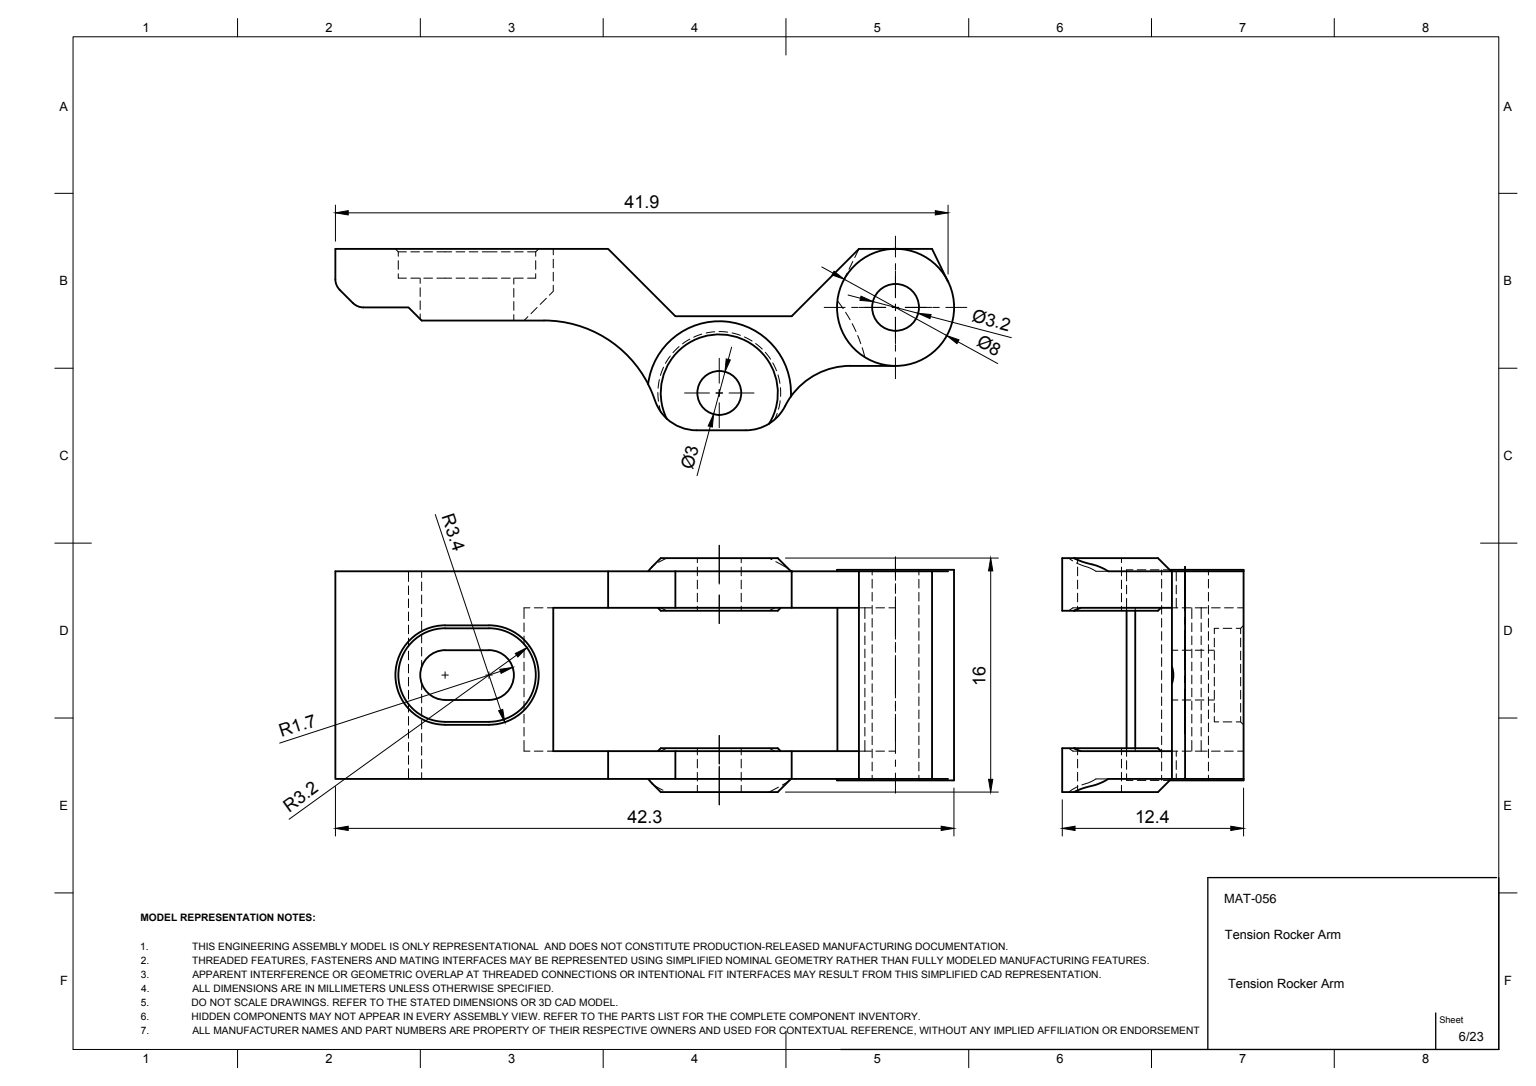
ISO-10303-21;
HEADER;
/* Generated by software containing ST-Developer
 * from STEP Tools, Inc. (www.steptools.com) 
 */

FILE_DESCRIPTION(
/* description */ (''),
/* implementation_level */ '2;1');

FILE_NAME(
/* name */ 'Tension Rocker Arm.step',
/* time_stamp */ '2026-10-28T16:47:13+01:00',
/* author */ (''),
/* organization */ (''),
/* preprocessor_version */ 'ST-DEVELOPER v20.2',
/* originating_system */ 'Autodesk Translation Framework v15.17.0.0',
/* authorisation */ '');

FILE_SCHEMA (('AUTOMOTIVE_DESIGN { 1 0 10303 214 3 1 1 }'));
ENDSEC;

DATA;
#10=MECHANICAL_DESIGN_GEOMETRIC_PRESENTATION_REPRESENTATION('',(#4571),#459242);
#185=ELLIPSE('',#97153,2.40416305603427,1.7);
#4408=SHAPE_REPRESENTATION_RELATIONSHIP('SRR','None',#459333,#4429);
#4429=ADVANCED_BREP_SHAPE_REPRESENTATION('',(#4451),#459222);
#4451=MANIFOLD_SOLID_BREP('Rocker',#94629);
#4571=STYLED_ITEM('',(#459519),#4451);
#4702=CONICAL_SURFACE('',#97156,3.3,0.785398163397448);
#4703=CONICAL_SURFACE('',#97159,3.3,0.785398163397448);
#4704=CONICAL_SURFACE('',#97173,4.45,0.785398163397448);
#4705=CONICAL_SURFACE('',#97175,4.45,0.785398163397449);
#4706=CONICAL_SURFACE('',#97185,4.1,0.785398163397445);
#4707=CONICAL_SURFACE('',#97187,4.1,0.785398163397445);
#5162=FACE_BOUND('',#13230,.T.);
#5163=FACE_BOUND('',#13257,.T.);
#5164=FACE_BOUND('',#13264,.T.);
#5165=FACE_BOUND('',#13266,.T.);
#5166=FACE_BOUND('',#13270,.T.);
#5167=FACE_BOUND('',#13272,.T.);
#5168=FACE_BOUND('',#13278,.T.);
#5169=FACE_BOUND('',#13281,.T.);
#5547=PLANE('',#97094);
#5548=PLANE('',#97095);
#5549=PLANE('',#97096);
#5550=PLANE('',#97103);
#5551=PLANE('',#97112);
#5552=PLANE('',#97113);
#5553=PLANE('',#97122);
#5554=PLANE('',#97123);
#5555=PLANE('',#97127);
#5556=PLANE('',#97130);
#5557=PLANE('',#97131);
#5558=PLANE('',#97134);
#5559=PLANE('',#97136);
#5560=PLANE('',#97137);
#5561=PLANE('',#97138);
#5562=PLANE('',#97139);
#5563=PLANE('',#97143);
#5564=PLANE('',#97144);
#5565=PLANE('',#97151);
#5566=PLANE('',#97152);
#5567=PLANE('',#97158);
#5568=PLANE('',#97161);
#5569=PLANE('',#97162);
#5570=PLANE('',#97165);
#5571=PLANE('',#97168);
#5572=PLANE('',#97170);
#5573=PLANE('',#97171);
#5574=PLANE('',#97177);
#5575=PLANE('',#97181);
#5576=PLANE('',#97189);
#5577=PLANE('',#97193);
#5578=PLANE('',#97199);
#5579=PLANE('',#97201);
#5580=PLANE('',#97204);
#5581=PLANE('',#97206);
#5582=PLANE('',#97209);
#5583=PLANE('',#97211);
#5584=PLANE('',#97212);
#5585=PLANE('',#97218);
#5586=PLANE('',#97219);
#7364=FACE_OUTER_BOUND('',#13221,.T.);
#7365=FACE_OUTER_BOUND('',#13222,.T.);
#7366=FACE_OUTER_BOUND('',#13223,.T.);
#7367=FACE_OUTER_BOUND('',#13224,.T.);
#7368=FACE_OUTER_BOUND('',#13225,.T.);
#7369=FACE_OUTER_BOUND('',#13226,.T.);
#7370=FACE_OUTER_BOUND('',#13227,.T.);
#7371=FACE_OUTER_BOUND('',#13228,.T.);
#7372=FACE_OUTER_BOUND('',#13229,.T.);
#7373=FACE_OUTER_BOUND('',#13231,.T.);
#7374=FACE_OUTER_BOUND('',#13232,.T.);
#7375=FACE_OUTER_BOUND('',#13233,.T.);
#7376=FACE_OUTER_BOUND('',#13234,.T.);
#7377=FACE_OUTER_BOUND('',#13235,.T.);
#7378=FACE_OUTER_BOUND('',#13236,.T.);
#7379=FACE_OUTER_BOUND('',#13237,.T.);
#7380=FACE_OUTER_BOUND('',#13238,.T.);
#7381=FACE_OUTER_BOUND('',#13239,.T.);
#7382=FACE_OUTER_BOUND('',#13240,.T.);
#7383=FACE_OUTER_BOUND('',#13241,.T.);
#7384=FACE_OUTER_BOUND('',#13242,.T.);
#7385=FACE_OUTER_BOUND('',#13243,.T.);
#7386=FACE_OUTER_BOUND('',#13244,.T.);
#7387=FACE_OUTER_BOUND('',#13245,.T.);
#7388=FACE_OUTER_BOUND('',#13246,.T.);
#7389=FACE_OUTER_BOUND('',#13247,.T.);
#7390=FACE_OUTER_BOUND('',#13248,.T.);
#7391=FACE_OUTER_BOUND('',#13249,.T.);
#7392=FACE_OUTER_BOUND('',#13250,.T.);
#7393=FACE_OUTER_BOUND('',#13251,.T.);
#7394=FACE_OUTER_BOUND('',#13252,.T.);
#7395=FACE_OUTER_BOUND('',#13253,.T.);
#7396=FACE_OUTER_BOUND('',#13254,.T.);
#7397=FACE_OUTER_BOUND('',#13255,.T.);
#7398=FACE_OUTER_BOUND('',#13256,.T.);
#7399=FACE_OUTER_BOUND('',#13258,.T.);
#7400=FACE_OUTER_BOUND('',#13259,.T.);
#7401=FACE_OUTER_BOUND('',#13260,.T.);
#7402=FACE_OUTER_BOUND('',#13261,.T.);
#7403=FACE_OUTER_BOUND('',#13262,.T.);
#7404=FACE_OUTER_BOUND('',#13263,.T.);
#7405=FACE_OUTER_BOUND('',#13265,.T.);
#7406=FACE_OUTER_BOUND('',#13267,.T.);
#7407=FACE_OUTER_BOUND('',#13268,.T.);
#7408=FACE_OUTER_BOUND('',#13269,.T.);
#7409=FACE_OUTER_BOUND('',#13271,.T.);
#7410=FACE_OUTER_BOUND('',#13273,.T.);
#7411=FACE_OUTER_BOUND('',#13274,.T.);
#7412=FACE_OUTER_BOUND('',#13275,.T.);
#7413=FACE_OUTER_BOUND('',#13276,.T.);
#7414=FACE_OUTER_BOUND('',#13277,.T.);
#7415=FACE_OUTER_BOUND('',#13279,.T.);
#7416=FACE_OUTER_BOUND('',#13280,.T.);
#7417=FACE_OUTER_BOUND('',#13282,.T.);
#7418=FACE_OUTER_BOUND('',#13283,.T.);
#7419=FACE_OUTER_BOUND('',#13284,.T.);
#7420=FACE_OUTER_BOUND('',#13285,.T.);
#7421=FACE_OUTER_BOUND('',#13286,.T.);
#7422=FACE_OUTER_BOUND('',#13287,.T.);
#7423=FACE_OUTER_BOUND('',#13288,.T.);
#7424=FACE_OUTER_BOUND('',#13289,.T.);
#7425=FACE_OUTER_BOUND('',#13290,.T.);
#7426=FACE_OUTER_BOUND('',#13291,.T.);
#7427=FACE_OUTER_BOUND('',#13292,.T.);
#7428=FACE_OUTER_BOUND('',#13293,.T.);
#7429=FACE_OUTER_BOUND('',#13294,.T.);
#13221=EDGE_LOOP('',(#63426,#63427,#63428,#63429));
#13222=EDGE_LOOP('',(#63430,#63431,#63432,#63433));
#13223=EDGE_LOOP('',(#63434,#63435,#63436,#63437,#63438,#63439,#63440,#63441,
#63442,#63443,#63444,#63445,#63446,#63447,#63448,#63449,#63450));
#13224=EDGE_LOOP('',(#63451,#63452,#63453,#63454,#63455,#63456,#63457,#63458,
#63459,#63460,#63461,#63462,#63463,#63464,#63465,#63466,#63467));
#13225=EDGE_LOOP('',(#63468,#63469,#63470,#63471));
#13226=EDGE_LOOP('',(#63472,#63473,#63474,#63475,#63476,#63477,#63478,#63479,
#63480,#63481,#63482,#63483,#63484,#63485,#63486,#63487,#63488));
#13227=EDGE_LOOP('',(#63489,#63490,#63491,#63492));
#13228=EDGE_LOOP('',(#63493,#63494,#63495,#63496,#63497,#63498,#63499,#63500,
#63501,#63502,#63503,#63504,#63505,#63506));
#13229=EDGE_LOOP('',(#63507,#63508,#63509,#63510,#63511,#63512,#63513,#63514));
#13230=EDGE_LOOP('',(#63515,#63516,#63517,#63518));
#13231=EDGE_LOOP('',(#63519,#63520,#63521,#63522));
#13232=EDGE_LOOP('',(#63523,#63524,#63525,#63526));
#13233=EDGE_LOOP('',(#63527,#63528,#63529,#63530,#63531));
#13234=EDGE_LOOP('',(#63532,#63533,#63534,#63535));
#13235=EDGE_LOOP('',(#63536,#63537,#63538,#63539));
#13236=EDGE_LOOP('',(#63540,#63541,#63542,#63543));
#13237=EDGE_LOOP('',(#63544,#63545,#63546,#63547));
#13238=EDGE_LOOP('',(#63548,#63549,#63550,#63551));
#13239=EDGE_LOOP('',(#63552,#63553,#63554,#63555));
#13240=EDGE_LOOP('',(#63556,#63557,#63558,#63559,#63560,#63561,#63562,#63563,
#63564,#63565));
#13241=EDGE_LOOP('',(#63566,#63567,#63568,#63569));
#13242=EDGE_LOOP('',(#63570,#63571,#63572,#63573));
#13243=EDGE_LOOP('',(#63574,#63575,#63576,#63577,#63578,#63579,#63580,#63581,
#63582,#63583,#63584,#63585,#63586,#63587,#63588,#63589,#63590));
#13244=EDGE_LOOP('',(#63591,#63592,#63593,#63594));
#13245=EDGE_LOOP('',(#63595,#63596,#63597,#63598));
#13246=EDGE_LOOP('',(#63599,#63600,#63601,#63602,#63603,#63604));
#13247=EDGE_LOOP('',(#63605,#63606,#63607,#63608,#63609,#63610));
#13248=EDGE_LOOP('',(#63611,#63612,#63613,#63614));
#13249=EDGE_LOOP('',(#63615,#63616,#63617,#63618));
#13250=EDGE_LOOP('',(#63619,#63620,#63621,#63622));
#13251=EDGE_LOOP('',(#63623,#63624,#63625,#63626));
#13252=EDGE_LOOP('',(#63627,#63628,#63629,#63630));
#13253=EDGE_LOOP('',(#63631,#63632,#63633,#63634));
#13254=EDGE_LOOP('',(#63635,#63636,#63637,#63638));
#13255=EDGE_LOOP('',(#63639,#63640,#63641,#63642));
#13256=EDGE_LOOP('',(#63643,#63644,#63645,#63646));
#13257=EDGE_LOOP('',(#63647,#63648,#63649,#63650));
#13258=EDGE_LOOP('',(#63651,#63652,#63653,#63654));
#13259=EDGE_LOOP('',(#63655,#63656,#63657,#63658));
#13260=EDGE_LOOP('',(#63659,#63660,#63661,#63662));
#13261=EDGE_LOOP('',(#63663,#63664,#63665,#63666,#63667,#63668));
#13262=EDGE_LOOP('',(#63669,#63670,#63671,#63672,#63673,#63674));
#13263=EDGE_LOOP('',(#63675,#63676,#63677,#63678));
#13264=EDGE_LOOP('',(#63679));
#13265=EDGE_LOOP('',(#63680,#63681,#63682,#63683));
#13266=EDGE_LOOP('',(#63684));
#13267=EDGE_LOOP('',(#63685,#63686,#63687,#63688));
#13268=EDGE_LOOP('',(#63689,#63690,#63691,#63692));
#13269=EDGE_LOOP('',(#63693,#63694,#63695,#63696));
#13270=EDGE_LOOP('',(#63697));
#13271=EDGE_LOOP('',(#63698,#63699,#63700,#63701));
#13272=EDGE_LOOP('',(#63702));
#13273=EDGE_LOOP('',(#63703,#63704,#63705,#63706,#63707));
#13274=EDGE_LOOP('',(#63708,#63709,#63710,#63711,#63712,#63713,#63714));
#13275=EDGE_LOOP('',(#63715,#63716,#63717,#63718));
#13276=EDGE_LOOP('',(#63719,#63720,#63721,#63722,#63723,#63724,#63725));
#13277=EDGE_LOOP('',(#63726));
#13278=EDGE_LOOP('',(#63727));
#13279=EDGE_LOOP('',(#63728,#63729,#63730));
#13280=EDGE_LOOP('',(#63731));
#13281=EDGE_LOOP('',(#63732));
#13282=EDGE_LOOP('',(#63733,#63734,#63735));
#13283=EDGE_LOOP('',(#63736,#63737,#63738,#63739));
#13284=EDGE_LOOP('',(#63740,#63741,#63742,#63743));
#13285=EDGE_LOOP('',(#63744,#63745,#63746,#63747,#63748));
#13286=EDGE_LOOP('',(#63749,#63750,#63751,#63752,#63753));
#13287=EDGE_LOOP('',(#63754,#63755,#63756,#63757,#63758,#63759,#63760));
#13288=EDGE_LOOP('',(#63761,#63762,#63763,#63764));
#13289=EDGE_LOOP('',(#63765,#63766,#63767,#63768,#63769,#63770,#63771));
#13290=EDGE_LOOP('',(#63772,#63773,#63774,#63775));
#13291=EDGE_LOOP('',(#63776,#63777,#63778,#63779));
#13292=EDGE_LOOP('',(#63780,#63781,#63782,#63783));
#13293=EDGE_LOOP('',(#63784,#63785,#63786,#63787));
#13294=EDGE_LOOP('',(#63788,#63789,#63790,#63791,#63792,#63793,#63794,#63795,
#63796,#63797,#63798,#63799,#63800,#63801,#63802,#63803,#63804,#63805));
#19394=CIRCLE('',#97097,4.);
#19395=CIRCLE('',#97098,5.);
#19396=CIRCLE('',#97099,4.9);
#19397=CIRCLE('',#97100,8.);
#19398=CIRCLE('',#97101,1.);
#19399=CIRCLE('',#97102,1.);
#19400=CIRCLE('',#97104,4.);
#19401=CIRCLE('',#97105,10.25);
#19402=CIRCLE('',#97106,4.);
#19403=CIRCLE('',#97107,5.);
#19404=CIRCLE('',#97108,3.);
#19405=CIRCLE('',#97109,4.2);
#19406=CIRCLE('',#97110,3.);
#19407=CIRCLE('',#97111,8.);
#19408=CIRCLE('',#97114,8.);
#19409=CIRCLE('',#97115,3.);
#19410=CIRCLE('',#97116,4.2);
#19411=CIRCLE('',#97117,3.);
#19412=CIRCLE('',#97118,5.);
#19413=CIRCLE('',#97119,4.);
#19414=CIRCLE('',#97120,10.25);
#19415=CIRCLE('',#97121,4.);
#19416=CIRCLE('',#97124,1.7);
#19417=CIRCLE('',#97125,1.7);
#19418=CIRCLE('',#97126,1.7);
#19419=CIRCLE('',#97128,3.4);
#19420=CIRCLE('',#97129,3.4);
#19421=CIRCLE('',#97140,4.);
#19422=CIRCLE('',#97142,1.);
#19423=CIRCLE('',#97145,1.);
#19424=CIRCLE('',#97146,8.);
#19425=CIRCLE('',#97147,4.9);
#19426=CIRCLE('',#97148,5.);
#19427=CIRCLE('',#97149,4.);
#19428=CIRCLE('',#97155,1.7);
#19429=CIRCLE('',#97157,3.2);
#19430=CIRCLE('',#97160,3.2);
#19431=CIRCLE('',#97164,3.2);
#19432=CIRCLE('',#97167,3.2);
#19433=CIRCLE('',#97169,1.7);
#19434=CIRCLE('',#97174,4.);
#19435=CIRCLE('',#97176,4.);
#19436=CIRCLE('',#97178,3.);
#19437=CIRCLE('',#97179,2.99999999999999);
#19438=CIRCLE('',#97180,1.5);
#19439=CIRCLE('',#97182,3.);
#19440=CIRCLE('',#97183,2.99999999999999);
#19441=CIRCLE('',#97184,1.5);
#19442=CIRCLE('',#97186,4.);
#19443=CIRCLE('',#97188,4.);
#19444=CIRCLE('',#97190,2.99999999999999);
#19445=CIRCLE('',#97191,3.);
#19446=CIRCLE('',#97192,1.5);
#19447=CIRCLE('',#97194,3.);
#19448=CIRCLE('',#97195,2.99999999999999);
#19449=CIRCLE('',#97196,1.5);
#19450=CIRCLE('',#97202,4.);
#19451=CIRCLE('',#97203,1.6);
#19452=CIRCLE('',#97205,4.);
#19453=CIRCLE('',#97207,4.);
#19454=CIRCLE('',#97208,1.6);
#19455=CIRCLE('',#97210,4.);
#23745=B_SPLINE_CURVE_WITH_KNOTS('',3,(#145559,#145560,#145561,#145562,
#145563,#145564),.UNSPECIFIED.,.F.,.F.,(4,2,4),(1.70223819819958,1.73108544940882,
1.82543924719591),.UNSPECIFIED.);
#23746=B_SPLINE_CURVE_WITH_KNOTS('',3,(#145675,#145676,#145677,#145678,
#145679,#145680),.UNSPECIFIED.,.F.,.F.,(4,2,4),(3.10863777787119,3.15979788758472,
3.18717384259103),.UNSPECIFIED.);
#23747=B_SPLINE_CURVE_WITH_KNOTS('',3,(#145682,#145683,#145684,#145685,
#145686,#145687),.UNSPECIFIED.,.F.,.F.,(4,2,4),(0.820560587522253,0.903541428390679,
0.986302965827679),.UNSPECIFIED.);
#23748=B_SPLINE_CURVE_WITH_KNOTS('',3,(#145690,#145691,#145692,#145693,
#145694,#145695,#145696,#145697),.UNSPECIFIED.,.F.,.F.,(4,2,2,4),(1.04408314569026,
1.07700516790035,1.159852876147,1.19188777117613),.UNSPECIFIED.);
#23749=B_SPLINE_CURVE_WITH_KNOTS('',3,(#145700,#145701,#145702,#145703,
#145704,#145705),.UNSPECIFIED.,.F.,.F.,(4,2,4),(0.461890211108374,0.489266166114685,
0.540426267783997),.UNSPECIFIED.);
#23750=B_SPLINE_CURVE_WITH_KNOTS('',3,(#145707,#145708,#145709,#145710,
#145711,#145712),.UNSPECIFIED.,.F.,.F.,(4,2,4),(1.94461759101078,2.03897139402255,
2.06781864523179),.UNSPECIFIED.);
#23751=B_SPLINE_CURVE_WITH_KNOTS('',3,(#145714,#145715,#145716,#145717,
#145718,#145719,#145720,#145721),.UNSPECIFIED.,.F.,.F.,(4,2,2,4),(0.734169017530397,
0.766203907566677,0.84905161581333,0.881973638023425),.UNSPECIFIED.);
#23752=B_SPLINE_CURVE_WITH_KNOTS('',3,(#145724,#145725,#145726,#145727,
#145728,#145729),.UNSPECIFIED.,.F.,.F.,(4,2,4),(0.991122094940072,1.07388363237707,
1.15686448098652),.UNSPECIFIED.);
#23753=B_SPLINE_CURVE_WITH_KNOTS('',3,(#145748,#145749,#145750,#145751),
 .UNSPECIFIED.,.F.,.F.,(4,4),(0.938179827022778,0.986302965827679),
 .UNSPECIFIED.);
#23754=B_SPLINE_CURVE_WITH_KNOTS('',3,(#145754,#145755,#145756,#145757,
#145758,#145759),.UNSPECIFIED.,.F.,.F.,(4,2,4),(1.04408314569026,1.07700516790035,
1.10576357261676),.UNSPECIFIED.);
#23755=B_SPLINE_CURVE_WITH_KNOTS('',3,(#145762,#145763,#145764,#145765,
#145766,#145767),.UNSPECIFIED.,.F.,.F.,(4,2,4),(0.820293211096921,0.84905161581333,
0.881973638023425),.UNSPECIFIED.);
#23756=B_SPLINE_CURVE_WITH_KNOTS('',3,(#145770,#145771,#145772,#145773),
 .UNSPECIFIED.,.F.,.F.,(4,4),(0.991122094940074,1.03924523374497),
 .UNSPECIFIED.);
#28169=LINE('',#145402,#31971);
#28170=LINE('',#145404,#31972);
#28171=LINE('',#145406,#31973);
#28172=LINE('',#145407,#31974);
#28173=LINE('',#145411,#31975);
#28174=LINE('',#145413,#31976);
#28175=LINE('',#145415,#31977);
#28176=LINE('',#145416,#31978);
#28177=LINE('',#145419,#31979);
#28178=LINE('',#145421,#31980);
#28179=LINE('',#145425,#31981);
#28180=LINE('',#145433,#31982);
#28181=LINE('',#145435,#31983);
#28182=LINE('',#145437,#31984);
#28183=LINE('',#145441,#31985);
#28184=LINE('',#145445,#31986);
#28185=LINE('',#145447,#31987);
#28186=LINE('',#145448,#31988);
#28187=LINE('',#145451,#31989);
#28188=LINE('',#145453,#31990);
#28189=LINE('',#145461,#31991);
#28190=LINE('',#145473,#31992);
#28191=LINE('',#145475,#31993);
#28192=LINE('',#145477,#31994);
#28193=LINE('',#145479,#31995);
#28194=LINE('',#145480,#31996);
#28195=LINE('',#145482,#31997);
#28196=LINE('',#145484,#31998);
#28197=LINE('',#145485,#31999);
#28198=LINE('',#145488,#32000);
#28199=LINE('',#145490,#32001);
#28200=LINE('',#145492,#32002);
#28201=LINE('',#145494,#32003);
#28202=LINE('',#145496,#32004);
#28203=LINE('',#145498,#32005);
#28204=LINE('',#145510,#32006);
#28205=LINE('',#145517,#32007);
#28206=LINE('',#145518,#32008);
#28207=LINE('',#145521,#32009);
#28208=LINE('',#145523,#32010);
#28209=LINE('',#145525,#32011);
#28210=LINE('',#145529,#32012);
#28211=LINE('',#145533,#32013);
#28212=LINE('',#145536,#32014);
#28213=LINE('',#145537,#32015);
#28214=LINE('',#145539,#32016);
#28215=LINE('',#145540,#32017);
#28216=LINE('',#145542,#32018);
#28217=LINE('',#145544,#32019);
#28218=LINE('',#145545,#32020);
#28219=LINE('',#145550,#32021);
#28220=LINE('',#145553,#32022);
#28221=LINE('',#145555,#32023);
#28222=LINE('',#145565,#32024);
#28223=LINE('',#145567,#32025);
#28224=LINE('',#145569,#32026);
#28225=LINE('',#145570,#32027);
#28226=LINE('',#145572,#32028);
#28227=LINE('',#145575,#32029);
#28228=LINE('',#145576,#32030);
#28229=LINE('',#145578,#32031);
#28230=LINE('',#145582,#32032);
#28231=LINE('',#145584,#32033);
#28232=LINE('',#145586,#32034);
#28233=LINE('',#145588,#32035);
#28234=LINE('',#145590,#32036);
#28235=LINE('',#145596,#32037);
#28236=LINE('',#145597,#32038);
#28237=LINE('',#145600,#32039);
#28238=LINE('',#145601,#32040);
#28239=LINE('',#145604,#32041);
#28240=LINE('',#145607,#32042);
#28241=LINE('',#145608,#32043);
#28242=LINE('',#145616,#32044);
#28243=LINE('',#145619,#32045);
#28244=LINE('',#145621,#32046);
#28245=LINE('',#145626,#32047);
#28246=LINE('',#145629,#32048);
#28247=LINE('',#145632,#32049);
#28248=LINE('',#145634,#32050);
#28249=LINE('',#145638,#32051);
#28250=LINE('',#145639,#32052);
#28251=LINE('',#145642,#32053);
#28252=LINE('',#145645,#32054);
#28253=LINE('',#145648,#32055);
#28254=LINE('',#145650,#32056);
#28255=LINE('',#145651,#32057);
#28256=LINE('',#145654,#32058);
#28257=LINE('',#145658,#32059);
#28258=LINE('',#145659,#32060);
#28259=LINE('',#145664,#32061);
#28260=LINE('',#145667,#32062);
#28261=LINE('',#145669,#32063);
#28262=LINE('',#145671,#32064);
#28263=LINE('',#145733,#32065);
#28264=LINE('',#145742,#32066);
#28265=LINE('',#145777,#32067);
#28266=LINE('',#145787,#32068);
#28267=LINE('',#145791,#32069);
#28268=LINE('',#145793,#32070);
#28269=LINE('',#145794,#32071);
#28270=LINE('',#145796,#32072);
#28271=LINE('',#145806,#32073);
#28272=LINE('',#145815,#32074);
#28273=LINE('',#145817,#32075);
#28274=LINE('',#145818,#32076);
#28275=LINE('',#145820,#32077);
#28276=LINE('',#145821,#32078);
#28277=LINE('',#145824,#32079);
#28278=LINE('',#145827,#32080);
#28279=LINE('',#145831,#32081);
#28280=LINE('',#145833,#32082);
#28281=LINE('',#145835,#32083);
#28282=LINE('',#145837,#32084);
#28283=LINE('',#145838,#32085);
#31971=VECTOR('',#111079,10.);
#31972=VECTOR('',#111080,10.);
#31973=VECTOR('',#111081,10.);
#31974=VECTOR('',#111082,10.);
#31975=VECTOR('',#111085,10.);
#31976=VECTOR('',#111086,10.);
#31977=VECTOR('',#111087,10.);
#31978=VECTOR('',#111088,10.);
#31979=VECTOR('',#111091,10.);
#31980=VECTOR('',#111092,10.);
#31981=VECTOR('',#111095,10.);
#31982=VECTOR('',#111102,10.);
#31983=VECTOR('',#111103,10.);
#31984=VECTOR('',#111104,10.);
#31985=VECTOR('',#111107,10.);
#31986=VECTOR('',#111110,10.);
#31987=VECTOR('',#111111,10.);
#31988=VECTOR('',#111112,10.);
#31989=VECTOR('',#111115,10.);
#31990=VECTOR('',#111116,10.);
#31991=VECTOR('',#111123,10.);
#31992=VECTOR('',#111134,10.);
#31993=VECTOR('',#111135,10.);
#31994=VECTOR('',#111136,10.);
#31995=VECTOR('',#111137,10.);
#31996=VECTOR('',#111138,10.);
#31997=VECTOR('',#111141,10.);
#31998=VECTOR('',#111142,10.);
#31999=VECTOR('',#111143,10.);
#32000=VECTOR('',#111146,10.);
#32001=VECTOR('',#111147,10.);
#32002=VECTOR('',#111148,10.);
#32003=VECTOR('',#111149,10.);
#32004=VECTOR('',#111150,10.);
#32005=VECTOR('',#111151,10.);
#32006=VECTOR('',#111162,10.);
#32007=VECTOR('',#111171,10.);
#32008=VECTOR('',#111172,10.);
#32009=VECTOR('',#111175,8.);
#32010=VECTOR('',#111176,10.);
#32011=VECTOR('',#111177,10.);
#32012=VECTOR('',#111180,10.);
#32013=VECTOR('',#111183,10.);
#32014=VECTOR('',#111186,10.);
#32015=VECTOR('',#111187,8.);
#32016=VECTOR('',#111190,10.);
#32017=VECTOR('',#111191,10.);
#32018=VECTOR('',#111192,10.);
#32019=VECTOR('',#111193,10.);
#32020=VECTOR('',#111194,10.);
#32021=VECTOR('',#111197,10.);
#32022=VECTOR('',#111200,10.);
#32023=VECTOR('',#111203,10.);
#32024=VECTOR('',#111208,10.);
#32025=VECTOR('',#111211,10.);
#32026=VECTOR('',#111214,5.);
#32027=VECTOR('',#111215,10.);
#32028=VECTOR('',#111218,10.);
#32029=VECTOR('',#111221,10.);
#32030=VECTOR('',#111222,10.);
#32031=VECTOR('',#111225,10.);
#32032=VECTOR('',#111230,10.);
#32033=VECTOR('',#111231,10.);
#32034=VECTOR('',#111232,10.);
#32035=VECTOR('',#111233,10.);
#32036=VECTOR('',#111234,10.);
#32037=VECTOR('',#111241,10.);
#32038=VECTOR('',#111242,10.);
#32039=VECTOR('',#111245,10.);
#32040=VECTOR('',#111246,10.);
#32041=VECTOR('',#111249,10.);
#32042=VECTOR('',#111252,10.);
#32043=VECTOR('',#111253,10.);
#32044=VECTOR('',#111260,10.);
#32045=VECTOR('',#111265,10.);
#32046=VECTOR('',#111268,10.);
#32047=VECTOR('',#111275,10.);
#32048=VECTOR('',#111278,10.);
#32049=VECTOR('',#111281,10.);
#32050=VECTOR('',#111282,10.);
#32051=VECTOR('',#111287,10.);
#32052=VECTOR('',#111288,10.);
#32053=VECTOR('',#111291,10.);
#32054=VECTOR('',#111296,10.);
#32055=VECTOR('',#111299,10.);
#32056=VECTOR('',#111300,10.);
#32057=VECTOR('',#111301,10.);
#32058=VECTOR('',#111304,10.);
#32059=VECTOR('',#111309,10.);
#32060=VECTOR('',#111310,10.);
#32061=VECTOR('',#111317,10.);
#32062=VECTOR('',#111320,10.);
#32063=VECTOR('',#111323,10.);
#32064=VECTOR('',#111326,10.);
#32065=VECTOR('',#111339,10.);
#32066=VECTOR('',#111350,10.);
#32067=VECTOR('',#111365,10.);
#32068=VECTOR('',#111378,10.);
#32069=VECTOR('',#111383,10.);
#32070=VECTOR('',#111386,10.);
#32071=VECTOR('',#111387,10.);
#32072=VECTOR('',#111390,10.);
#32073=VECTOR('',#111403,10.);
#32074=VECTOR('',#111414,10.);
#32075=VECTOR('',#111417,10.);
#32076=VECTOR('',#111418,5.);
#32077=VECTOR('',#111421,10.);
#32078=VECTOR('',#111422,10.);
#32079=VECTOR('',#111427,10.);
#32080=VECTOR('',#111432,1.5);
#32081=VECTOR('',#111439,10.);
#32082=VECTOR('',#111442,1.6);
#32083=VECTOR('',#111445,1.5);
#32084=VECTOR('',#111448,4.);
#32085=VECTOR('',#111449,4.);
#36364=VERTEX_POINT('',#145400);
#36365=VERTEX_POINT('',#145401);
#36366=VERTEX_POINT('',#145403);
#36367=VERTEX_POINT('',#145405);
#36368=VERTEX_POINT('',#145409);
#36369=VERTEX_POINT('',#145410);
#36370=VERTEX_POINT('',#145412);
#36371=VERTEX_POINT('',#145414);
#36372=VERTEX_POINT('',#145418);
#36373=VERTEX_POINT('',#145420);
#36374=VERTEX_POINT('',#145422);
#36375=VERTEX_POINT('',#145424);
#36376=VERTEX_POINT('',#145426);
#36377=VERTEX_POINT('',#145428);
#36378=VERTEX_POINT('',#145430);
#36379=VERTEX_POINT('',#145432);
#36380=VERTEX_POINT('',#145434);
#36381=VERTEX_POINT('',#145436);
#36382=VERTEX_POINT('',#145438);
#36383=VERTEX_POINT('',#145440);
#36384=VERTEX_POINT('',#145442);
#36385=VERTEX_POINT('',#145444);
#36386=VERTEX_POINT('',#145446);
#36387=VERTEX_POINT('',#145450);
#36388=VERTEX_POINT('',#145452);
#36389=VERTEX_POINT('',#145454);
#36390=VERTEX_POINT('',#145456);
#36391=VERTEX_POINT('',#145458);
#36392=VERTEX_POINT('',#145460);
#36393=VERTEX_POINT('',#145462);
#36394=VERTEX_POINT('',#145464);
#36395=VERTEX_POINT('',#145466);
#36396=VERTEX_POINT('',#145468);
#36397=VERTEX_POINT('',#145470);
#36398=VERTEX_POINT('',#145472);
#36399=VERTEX_POINT('',#145474);
#36400=VERTEX_POINT('',#145476);
#36401=VERTEX_POINT('',#145478);
#36402=VERTEX_POINT('',#145483);
#36403=VERTEX_POINT('',#145487);
#36404=VERTEX_POINT('',#145489);
#36405=VERTEX_POINT('',#145491);
#36406=VERTEX_POINT('',#145493);
#36407=VERTEX_POINT('',#145495);
#36408=VERTEX_POINT('',#145497);
#36409=VERTEX_POINT('',#145499);
#36410=VERTEX_POINT('',#145501);
#36411=VERTEX_POINT('',#145503);
#36412=VERTEX_POINT('',#145505);
#36413=VERTEX_POINT('',#145507);
#36414=VERTEX_POINT('',#145509);
#36415=VERTEX_POINT('',#145511);
#36416=VERTEX_POINT('',#145513);
#36417=VERTEX_POINT('',#145520);
#36418=VERTEX_POINT('',#145522);
#36419=VERTEX_POINT('',#145524);
#36420=VERTEX_POINT('',#145526);
#36421=VERTEX_POINT('',#145528);
#36422=VERTEX_POINT('',#145530);
#36423=VERTEX_POINT('',#145532);
#36424=VERTEX_POINT('',#145534);
#36425=VERTEX_POINT('',#145541);
#36426=VERTEX_POINT('',#145543);
#36427=VERTEX_POINT('',#145546);
#36428=VERTEX_POINT('',#145547);
#36429=VERTEX_POINT('',#145549);
#36430=VERTEX_POINT('',#145551);
#36431=VERTEX_POINT('',#145558);
#36432=VERTEX_POINT('',#145574);
#36433=VERTEX_POINT('',#145581);
#36434=VERTEX_POINT('',#145583);
#36435=VERTEX_POINT('',#145585);
#36436=VERTEX_POINT('',#145587);
#36437=VERTEX_POINT('',#145589);
#36438=VERTEX_POINT('',#145593);
#36439=VERTEX_POINT('',#145594);
#36440=VERTEX_POINT('',#145599);
#36441=VERTEX_POINT('',#145603);
#36442=VERTEX_POINT('',#145606);
#36443=VERTEX_POINT('',#145609);
#36444=VERTEX_POINT('',#145611);
#36445=VERTEX_POINT('',#145613);
#36446=VERTEX_POINT('',#145615);
#36447=VERTEX_POINT('',#145625);
#36448=VERTEX_POINT('',#145627);
#36449=VERTEX_POINT('',#145631);
#36450=VERTEX_POINT('',#145633);
#36451=VERTEX_POINT('',#145637);
#36452=VERTEX_POINT('',#145641);
#36453=VERTEX_POINT('',#145647);
#36454=VERTEX_POINT('',#145649);
#36455=VERTEX_POINT('',#145653);
#36456=VERTEX_POINT('',#145657);
#36457=VERTEX_POINT('',#145663);
#36458=VERTEX_POINT('',#145665);
#36459=VERTEX_POINT('',#145674);
#36460=VERTEX_POINT('',#145681);
#36461=VERTEX_POINT('',#145688);
#36462=VERTEX_POINT('',#145699);
#36463=VERTEX_POINT('',#145706);
#36464=VERTEX_POINT('',#145713);
#36465=VERTEX_POINT('',#145722);
#36466=VERTEX_POINT('',#145731);
#36467=VERTEX_POINT('',#145732);
#36468=VERTEX_POINT('',#145736);
#36469=VERTEX_POINT('',#145739);
#36470=VERTEX_POINT('',#145741);
#36471=VERTEX_POINT('',#145744);
#36472=VERTEX_POINT('',#145747);
#36473=VERTEX_POINT('',#145752);
#36474=VERTEX_POINT('',#145761);
#36475=VERTEX_POINT('',#145768);
#36476=VERTEX_POINT('',#145775);
#36477=VERTEX_POINT('',#145776);
#36478=VERTEX_POINT('',#145780);
#36479=VERTEX_POINT('',#145783);
#36480=VERTEX_POINT('',#145785);
#36481=VERTEX_POINT('',#145788);
#36482=VERTEX_POINT('',#145799);
#36483=VERTEX_POINT('',#145801);
#36484=VERTEX_POINT('',#145804);
#36485=VERTEX_POINT('',#145808);
#36486=VERTEX_POINT('',#145810);
#36487=VERTEX_POINT('',#145813);
#46215=EDGE_CURVE('',#36364,#36365,#28169,.T.);
#46216=EDGE_CURVE('',#36366,#36364,#28170,.T.);
#46217=EDGE_CURVE('',#36367,#36366,#28171,.T.);
#46218=EDGE_CURVE('',#36365,#36367,#28172,.T.);
#46219=EDGE_CURVE('',#36368,#36369,#28173,.T.);
#46220=EDGE_CURVE('',#36370,#36368,#28174,.T.);
#46221=EDGE_CURVE('',#36371,#36370,#28175,.T.);
#46222=EDGE_CURVE('',#36369,#36371,#28176,.T.);
#46223=EDGE_CURVE('',#36372,#36367,#28177,.T.);
#46224=EDGE_CURVE('',#36373,#36366,#28178,.T.);
#46225=EDGE_CURVE('',#36373,#36374,#19394,.T.);
#46226=EDGE_CURVE('',#36374,#36375,#28179,.T.);
#46227=EDGE_CURVE('',#36375,#36376,#19395,.F.);
#46228=EDGE_CURVE('',#36377,#36376,#19396,.T.);
#46229=EDGE_CURVE('',#36377,#36378,#19397,.F.);
#46230=EDGE_CURVE('',#36378,#36379,#28180,.T.);
#46231=EDGE_CURVE('',#36379,#36380,#28181,.T.);
#46232=EDGE_CURVE('',#36380,#36381,#28182,.T.);
#46233=EDGE_CURVE('',#36382,#36381,#19398,.T.);
#46234=EDGE_CURVE('',#36383,#36382,#28183,.T.);
#46235=EDGE_CURVE('',#36384,#36383,#19399,.T.);
#46236=EDGE_CURVE('',#36384,#36385,#28184,.T.);
#46237=EDGE_CURVE('',#36386,#36385,#28185,.T.);
#46238=EDGE_CURVE('',#36386,#36372,#28186,.T.);
#46239=EDGE_CURVE('',#36387,#36368,#28187,.T.);
#46240=EDGE_CURVE('',#36369,#36388,#28188,.T.);
#46241=EDGE_CURVE('',#36389,#36388,#19400,.T.);
#46242=EDGE_CURVE('',#36390,#36389,#19401,.T.);
#46243=EDGE_CURVE('',#36391,#36390,#19402,.T.);
#46244=EDGE_CURVE('',#36392,#36391,#28189,.T.);
#46245=EDGE_CURVE('',#36393,#36392,#19403,.T.);
#46246=EDGE_CURVE('',#36394,#36393,#19404,.T.);
#46247=EDGE_CURVE('',#36395,#36394,#19405,.T.);
#46248=EDGE_CURVE('',#36396,#36395,#19406,.T.);
#46249=EDGE_CURVE('',#36397,#36396,#19407,.T.);
#46250=EDGE_CURVE('',#36397,#36398,#28190,.T.);
#46251=EDGE_CURVE('',#36398,#36399,#28191,.T.);
#46252=EDGE_CURVE('',#36399,#36400,#28192,.T.);
#46253=EDGE_CURVE('',#36401,#36400,#28193,.T.);
#46254=EDGE_CURVE('',#36387,#36401,#28194,.T.);
#46255=EDGE_CURVE('',#36364,#36369,#28195,.T.);
#46256=EDGE_CURVE('',#36364,#36402,#28196,.T.);
#46257=EDGE_CURVE('',#36402,#36388,#28197,.T.);
#46258=EDGE_CURVE('',#36365,#36403,#28198,.T.);
#46259=EDGE_CURVE('',#36404,#36403,#28199,.T.);
#46260=EDGE_CURVE('',#36405,#36404,#28200,.T.);
#46261=EDGE_CURVE('',#36405,#36406,#28201,.T.);
#46262=EDGE_CURVE('',#36407,#36406,#28202,.F.);
#46263=EDGE_CURVE('',#36407,#36408,#28203,.T.);
#46264=EDGE_CURVE('',#36409,#36408,#19408,.T.);
#46265=EDGE_CURVE('',#36410,#36409,#19409,.T.);
#46266=EDGE_CURVE('',#36411,#36410,#19410,.T.);
#46267=EDGE_CURVE('',#36412,#36411,#19411,.T.);
#46268=EDGE_CURVE('',#36413,#36412,#19412,.T.);
#46269=EDGE_CURVE('',#36414,#36413,#28204,.T.);
#46270=EDGE_CURVE('',#36415,#36414,#19413,.T.);
#46271=EDGE_CURVE('',#36416,#36415,#19414,.T.);
#46272=EDGE_CURVE('',#36402,#36416,#19415,.T.);
#46273=EDGE_CURVE('',#36406,#36399,#28205,.T.);
#46274=EDGE_CURVE('',#36398,#36407,#28206,.T.);
#46275=EDGE_CURVE('',#36417,#36397,#28207,.T.);
#46276=EDGE_CURVE('',#36418,#36417,#28208,.F.);
#46277=EDGE_CURVE('',#36418,#36419,#28209,.T.);
#46278=EDGE_CURVE('',#36419,#36420,#19416,.T.);
#46279=EDGE_CURVE('',#36420,#36421,#28210,.T.);
#46280=EDGE_CURVE('',#36421,#36422,#19417,.T.);
#46281=EDGE_CURVE('',#36422,#36423,#28211,.T.);
#46282=EDGE_CURVE('',#36423,#36424,#19418,.T.);
#46283=EDGE_CURVE('',#36424,#36379,#28212,.T.);
#46284=EDGE_CURVE('',#36408,#36378,#28213,.T.);
#46285=EDGE_CURVE('',#36400,#36405,#28214,.T.);
#46286=EDGE_CURVE('',#36404,#36386,#28215,.T.);
#46287=EDGE_CURVE('',#36385,#36425,#28216,.F.);
#46288=EDGE_CURVE('',#36426,#36425,#28217,.F.);
#46289=EDGE_CURVE('',#36426,#36401,#28218,.T.);
#46290=EDGE_CURVE('',#36427,#36428,#19419,.T.);
#46291=EDGE_CURVE('',#36429,#36427,#28219,.T.);
#46292=EDGE_CURVE('',#36430,#36429,#19420,.T.);
#46293=EDGE_CURVE('',#36428,#36430,#28220,.T.);
#46294=EDGE_CURVE('',#36403,#36372,#28221,.T.);
#46295=EDGE_CURVE('',#36377,#36431,#23745,.T.);
#46296=EDGE_CURVE('',#36409,#36431,#28222,.T.);
#46297=EDGE_CURVE('',#36389,#36416,#28223,.T.);
#46298=EDGE_CURVE('',#36375,#36413,#28224,.T.);
#46299=EDGE_CURVE('',#36374,#36414,#28225,.T.);
#46300=EDGE_CURVE('',#36415,#36390,#28226,.T.);
#46301=EDGE_CURVE('',#36432,#36426,#28227,.T.);
#46302=EDGE_CURVE('',#36432,#36387,#28228,.T.);
#46303=EDGE_CURVE('',#36370,#36432,#28229,.T.);
#46304=EDGE_CURVE('',#36433,#36371,#28230,.F.);
#46305=EDGE_CURVE('',#36434,#36433,#28231,.F.);
#46306=EDGE_CURVE('',#36435,#36434,#28232,.F.);
#46307=EDGE_CURVE('',#36436,#36435,#28233,.T.);
#46308=EDGE_CURVE('',#36436,#36437,#28234,.T.);
#46309=EDGE_CURVE('',#36437,#36373,#19421,.T.);
#46310=EDGE_CURVE('',#36438,#36439,#19422,.T.);
#46311=EDGE_CURVE('',#36439,#36382,#28235,.T.);
#46312=EDGE_CURVE('',#36381,#36438,#28236,.T.);
#46313=EDGE_CURVE('',#36439,#36440,#28237,.T.);
#46314=EDGE_CURVE('',#36383,#36440,#28238,.T.);
#46315=EDGE_CURVE('',#36425,#36441,#28239,.T.);
#46316=EDGE_CURVE('',#36440,#36441,#19423,.T.);
#46317=EDGE_CURVE('',#36438,#36442,#28240,.T.);
#46318=EDGE_CURVE('',#36442,#36418,#28241,.T.);
#46319=EDGE_CURVE('',#36443,#36417,#19424,.T.);
#46320=EDGE_CURVE('',#36444,#36443,#19425,.T.);
#46321=EDGE_CURVE('',#36445,#36444,#19426,.T.);
#46322=EDGE_CURVE('',#36445,#36446,#28242,.F.);
#46323=EDGE_CURVE('',#36446,#36433,#19427,.T.);
#46324=EDGE_CURVE('',#36441,#36384,#28243,.T.);
#46325=EDGE_CURVE('',#36442,#36380,#28244,.T.);
#46326=EDGE_CURVE('',#36419,#36424,#185,.T.);
#46327=EDGE_CURVE('',#36447,#36423,#28245,.T.);
#46328=EDGE_CURVE('',#36447,#36448,#19428,.T.);
#46329=EDGE_CURVE('',#36448,#36420,#28246,.T.);
#46330=EDGE_CURVE('',#36449,#36427,#28247,.T.);
#46331=EDGE_CURVE('',#36428,#36450,#28248,.T.);
#46332=EDGE_CURVE('',#36450,#36449,#19429,.T.);
#46333=EDGE_CURVE('',#36451,#36429,#28249,.T.);
#46334=EDGE_CURVE('',#36449,#36451,#28250,.T.);
#46335=EDGE_CURVE('',#36452,#36430,#28251,.T.);
#46336=EDGE_CURVE('',#36451,#36452,#19430,.T.);
#46337=EDGE_CURVE('',#36452,#36450,#28252,.T.);
#46338=EDGE_CURVE('',#36449,#36453,#28253,.T.);
#46339=EDGE_CURVE('',#36453,#36454,#28254,.T.);
#46340=EDGE_CURVE('',#36451,#36454,#28255,.T.);
#46341=EDGE_CURVE('',#36450,#36455,#28256,.T.);
#46342=EDGE_CURVE('',#36455,#36453,#19431,.T.);
#46343=EDGE_CURVE('',#36452,#36456,#28257,.T.);
#46344=EDGE_CURVE('',#36456,#36455,#28258,.T.);
#46345=EDGE_CURVE('',#36454,#36456,#19432,.T.);
#46346=EDGE_CURVE('',#36457,#36447,#28259,.T.);
#46347=EDGE_CURVE('',#36458,#36457,#19433,.T.);
#46348=EDGE_CURVE('',#36448,#36458,#28260,.T.);
#46349=EDGE_CURVE('',#36457,#36422,#28261,.T.);
#46350=EDGE_CURVE('',#36458,#36421,#28262,.T.);
#46351=EDGE_CURVE('',#36376,#36459,#23746,.F.);
#46352=EDGE_CURVE('',#36460,#36459,#23747,.F.);
#46353=EDGE_CURVE('',#36461,#36460,#19434,.T.);
#46354=EDGE_CURVE('',#36431,#36461,#23748,.F.);
#46355=EDGE_CURVE('',#36444,#36462,#23749,.T.);
#46356=EDGE_CURVE('',#36443,#36463,#23750,.F.);
#46357=EDGE_CURVE('',#36464,#36463,#23751,.F.);
#46358=EDGE_CURVE('',#36465,#36464,#19435,.T.);
#46359=EDGE_CURVE('',#36462,#36465,#23752,.F.);
#46360=EDGE_CURVE('',#36466,#36467,#28263,.T.);
#46361=EDGE_CURVE('',#36467,#36461,#19436,.T.);
#46362=EDGE_CURVE('',#36460,#36466,#19437,.T.);
#46363=EDGE_CURVE('',#36468,#36468,#19438,.T.);
#46364=EDGE_CURVE('',#36464,#36469,#19439,.T.);
#46365=EDGE_CURVE('',#36469,#36470,#28264,.T.);
#46366=EDGE_CURVE('',#36470,#36465,#19440,.T.);
#46367=EDGE_CURVE('',#36471,#36471,#19441,.T.);
#46368=EDGE_CURVE('',#36394,#36472,#23753,.T.);
#46369=EDGE_CURVE('',#36473,#36472,#19442,.T.);
#46370=EDGE_CURVE('',#36473,#36395,#23754,.T.);
#46371=EDGE_CURVE('',#36410,#36474,#23755,.T.);
#46372=EDGE_CURVE('',#36475,#36474,#19443,.T.);
#46373=EDGE_CURVE('',#36475,#36411,#23756,.T.);
#46374=EDGE_CURVE('',#36476,#36477,#28265,.T.);
#46375=EDGE_CURVE('',#36477,#36475,#19444,.T.);
#46376=EDGE_CURVE('',#36474,#36476,#19445,.T.);
#46377=EDGE_CURVE('',#36478,#36478,#19446,.T.);
#46378=EDGE_CURVE('',#36479,#36473,#19447,.T.);
#46379=EDGE_CURVE('',#36472,#36480,#19448,.T.);
#46380=EDGE_CURVE('',#36480,#36479,#28266,.T.);
#46381=EDGE_CURVE('',#36481,#36481,#19449,.T.);
#46382=EDGE_CURVE('',#36463,#36396,#28267,.F.);
#46383=EDGE_CURVE('',#36477,#36466,#28268,.T.);
#46384=EDGE_CURVE('',#36459,#36412,#28269,.T.);
#46385=EDGE_CURVE('',#36467,#36476,#28270,.T.);
#46386=EDGE_CURVE('',#36482,#36482,#19450,.T.);
#46387=EDGE_CURVE('',#36483,#36483,#19451,.T.);
#46388=EDGE_CURVE('',#36434,#36484,#19452,.T.);
#46389=EDGE_CURVE('',#36484,#36435,#28271,.F.);
#46390=EDGE_CURVE('',#36485,#36485,#19453,.T.);
#46391=EDGE_CURVE('',#36486,#36486,#19454,.T.);
#46392=EDGE_CURVE('',#36487,#36437,#19455,.T.);
#46393=EDGE_CURVE('',#36436,#36487,#28272,.T.);
#46394=EDGE_CURVE('',#36391,#36446,#28273,.T.);
#46395=EDGE_CURVE('',#36392,#36445,#28274,.T.);
#46396=EDGE_CURVE('',#36470,#36480,#28275,.T.);
#46397=EDGE_CURVE('',#36479,#36469,#28276,.T.);
#46398=EDGE_CURVE('',#36462,#36393,#28277,.F.);
#46399=EDGE_CURVE('',#36478,#36468,#28278,.T.);
#46400=EDGE_CURVE('',#36487,#36484,#28279,.T.);
#46401=EDGE_CURVE('',#36483,#36486,#28280,.T.);
#46402=EDGE_CURVE('',#36471,#36481,#28281,.T.);
#46403=EDGE_CURVE('',#36482,#36434,#28282,.T.);
#46404=EDGE_CURVE('',#36437,#36485,#28283,.T.);
#63426=ORIENTED_EDGE('',*,*,#46215,.F.);
#63427=ORIENTED_EDGE('',*,*,#46216,.F.);
#63428=ORIENTED_EDGE('',*,*,#46217,.F.);
#63429=ORIENTED_EDGE('',*,*,#46218,.F.);
#63430=ORIENTED_EDGE('',*,*,#46219,.F.);
#63431=ORIENTED_EDGE('',*,*,#46220,.F.);
#63432=ORIENTED_EDGE('',*,*,#46221,.F.);
#63433=ORIENTED_EDGE('',*,*,#46222,.F.);
#63434=ORIENTED_EDGE('',*,*,#46223,.T.);
#63435=ORIENTED_EDGE('',*,*,#46217,.T.);
#63436=ORIENTED_EDGE('',*,*,#46224,.F.);
#63437=ORIENTED_EDGE('',*,*,#46225,.T.);
#63438=ORIENTED_EDGE('',*,*,#46226,.T.);
#63439=ORIENTED_EDGE('',*,*,#46227,.T.);
#63440=ORIENTED_EDGE('',*,*,#46228,.F.);
#63441=ORIENTED_EDGE('',*,*,#46229,.T.);
#63442=ORIENTED_EDGE('',*,*,#46230,.T.);
#63443=ORIENTED_EDGE('',*,*,#46231,.T.);
#63444=ORIENTED_EDGE('',*,*,#46232,.T.);
#63445=ORIENTED_EDGE('',*,*,#46233,.F.);
#63446=ORIENTED_EDGE('',*,*,#46234,.F.);
#63447=ORIENTED_EDGE('',*,*,#46235,.F.);
#63448=ORIENTED_EDGE('',*,*,#46236,.T.);
#63449=ORIENTED_EDGE('',*,*,#46237,.F.);
#63450=ORIENTED_EDGE('',*,*,#46238,.T.);
#63451=ORIENTED_EDGE('',*,*,#46239,.T.);
#63452=ORIENTED_EDGE('',*,*,#46219,.T.);
#63453=ORIENTED_EDGE('',*,*,#46240,.T.);
#63454=ORIENTED_EDGE('',*,*,#46241,.F.);
#63455=ORIENTED_EDGE('',*,*,#46242,.F.);
#63456=ORIENTED_EDGE('',*,*,#46243,.F.);
#63457=ORIENTED_EDGE('',*,*,#46244,.F.);
#63458=ORIENTED_EDGE('',*,*,#46245,.F.);
#63459=ORIENTED_EDGE('',*,*,#46246,.F.);
#63460=ORIENTED_EDGE('',*,*,#46247,.F.);
#63461=ORIENTED_EDGE('',*,*,#46248,.F.);
#63462=ORIENTED_EDGE('',*,*,#46249,.F.);
#63463=ORIENTED_EDGE('',*,*,#46250,.T.);
#63464=ORIENTED_EDGE('',*,*,#46251,.T.);
#63465=ORIENTED_EDGE('',*,*,#46252,.T.);
#63466=ORIENTED_EDGE('',*,*,#46253,.F.);
#63467=ORIENTED_EDGE('',*,*,#46254,.F.);
#63468=ORIENTED_EDGE('',*,*,#46240,.F.);
#63469=ORIENTED_EDGE('',*,*,#46255,.F.);
#63470=ORIENTED_EDGE('',*,*,#46256,.T.);
#63471=ORIENTED_EDGE('',*,*,#46257,.T.);
#63472=ORIENTED_EDGE('',*,*,#46258,.T.);
#63473=ORIENTED_EDGE('',*,*,#46259,.F.);
#63474=ORIENTED_EDGE('',*,*,#46260,.F.);
#63475=ORIENTED_EDGE('',*,*,#46261,.T.);
#63476=ORIENTED_EDGE('',*,*,#46262,.F.);
#63477=ORIENTED_EDGE('',*,*,#46263,.T.);
#63478=ORIENTED_EDGE('',*,*,#46264,.F.);
#63479=ORIENTED_EDGE('',*,*,#46265,.F.);
#63480=ORIENTED_EDGE('',*,*,#46266,.F.);
#63481=ORIENTED_EDGE('',*,*,#46267,.F.);
#63482=ORIENTED_EDGE('',*,*,#46268,.F.);
#63483=ORIENTED_EDGE('',*,*,#46269,.F.);
#63484=ORIENTED_EDGE('',*,*,#46270,.F.);
#63485=ORIENTED_EDGE('',*,*,#46271,.F.);
#63486=ORIENTED_EDGE('',*,*,#46272,.F.);
#63487=ORIENTED_EDGE('',*,*,#46256,.F.);
#63488=ORIENTED_EDGE('',*,*,#46215,.T.);
#63489=ORIENTED_EDGE('',*,*,#46262,.T.);
#63490=ORIENTED_EDGE('',*,*,#46273,.T.);
#63491=ORIENTED_EDGE('',*,*,#46251,.F.);
#63492=ORIENTED_EDGE('',*,*,#46274,.T.);
#63493=ORIENTED_EDGE('',*,*,#46263,.F.);
#63494=ORIENTED_EDGE('',*,*,#46274,.F.);
#63495=ORIENTED_EDGE('',*,*,#46250,.F.);
#63496=ORIENTED_EDGE('',*,*,#46275,.F.);
#63497=ORIENTED_EDGE('',*,*,#46276,.F.);
#63498=ORIENTED_EDGE('',*,*,#46277,.T.);
#63499=ORIENTED_EDGE('',*,*,#46278,.T.);
#63500=ORIENTED_EDGE('',*,*,#46279,.T.);
#63501=ORIENTED_EDGE('',*,*,#46280,.T.);
#63502=ORIENTED_EDGE('',*,*,#46281,.T.);
#63503=ORIENTED_EDGE('',*,*,#46282,.T.);
#63504=ORIENTED_EDGE('',*,*,#46283,.T.);
#63505=ORIENTED_EDGE('',*,*,#46230,.F.);
#63506=ORIENTED_EDGE('',*,*,#46284,.F.);
#63507=ORIENTED_EDGE('',*,*,#46253,.T.);
#63508=ORIENTED_EDGE('',*,*,#46285,.T.);
#63509=ORIENTED_EDGE('',*,*,#46260,.T.);
#63510=ORIENTED_EDGE('',*,*,#46286,.T.);
#63511=ORIENTED_EDGE('',*,*,#46237,.T.);
#63512=ORIENTED_EDGE('',*,*,#46287,.T.);
#63513=ORIENTED_EDGE('',*,*,#46288,.F.);
#63514=ORIENTED_EDGE('',*,*,#46289,.T.);
#63515=ORIENTED_EDGE('',*,*,#46290,.F.);
#63516=ORIENTED_EDGE('',*,*,#46291,.F.);
#63517=ORIENTED_EDGE('',*,*,#46292,.F.);
#63518=ORIENTED_EDGE('',*,*,#46293,.F.);
#63519=ORIENTED_EDGE('',*,*,#46259,.T.);
#63520=ORIENTED_EDGE('',*,*,#46294,.T.);
#63521=ORIENTED_EDGE('',*,*,#46238,.F.);
#63522=ORIENTED_EDGE('',*,*,#46286,.F.);
#63523=ORIENTED_EDGE('',*,*,#46273,.F.);
#63524=ORIENTED_EDGE('',*,*,#46261,.F.);
#63525=ORIENTED_EDGE('',*,*,#46285,.F.);
#63526=ORIENTED_EDGE('',*,*,#46252,.F.);
#63527=ORIENTED_EDGE('',*,*,#46264,.T.);
#63528=ORIENTED_EDGE('',*,*,#46284,.T.);
#63529=ORIENTED_EDGE('',*,*,#46229,.F.);
#63530=ORIENTED_EDGE('',*,*,#46295,.T.);
#63531=ORIENTED_EDGE('',*,*,#46296,.F.);
#63532=ORIENTED_EDGE('',*,*,#46257,.F.);
#63533=ORIENTED_EDGE('',*,*,#46272,.T.);
#63534=ORIENTED_EDGE('',*,*,#46297,.F.);
#63535=ORIENTED_EDGE('',*,*,#46241,.T.);
#63536=ORIENTED_EDGE('',*,*,#46269,.T.);
#63537=ORIENTED_EDGE('',*,*,#46298,.F.);
#63538=ORIENTED_EDGE('',*,*,#46226,.F.);
#63539=ORIENTED_EDGE('',*,*,#46299,.T.);
#63540=ORIENTED_EDGE('',*,*,#46297,.T.);
#63541=ORIENTED_EDGE('',*,*,#46271,.T.);
#63542=ORIENTED_EDGE('',*,*,#46300,.T.);
#63543=ORIENTED_EDGE('',*,*,#46242,.T.);
#63544=ORIENTED_EDGE('',*,*,#46254,.T.);
#63545=ORIENTED_EDGE('',*,*,#46289,.F.);
#63546=ORIENTED_EDGE('',*,*,#46301,.F.);
#63547=ORIENTED_EDGE('',*,*,#46302,.T.);
#63548=ORIENTED_EDGE('',*,*,#46303,.F.);
#63549=ORIENTED_EDGE('',*,*,#46220,.T.);
#63550=ORIENTED_EDGE('',*,*,#46239,.F.);
#63551=ORIENTED_EDGE('',*,*,#46302,.F.);
#63552=ORIENTED_EDGE('',*,*,#46223,.F.);
#63553=ORIENTED_EDGE('',*,*,#46294,.F.);
#63554=ORIENTED_EDGE('',*,*,#46258,.F.);
#63555=ORIENTED_EDGE('',*,*,#46218,.T.);
#63556=ORIENTED_EDGE('',*,*,#46222,.T.);
#63557=ORIENTED_EDGE('',*,*,#46304,.F.);
#63558=ORIENTED_EDGE('',*,*,#46305,.F.);
#63559=ORIENTED_EDGE('',*,*,#46306,.F.);
#63560=ORIENTED_EDGE('',*,*,#46307,.F.);
#63561=ORIENTED_EDGE('',*,*,#46308,.T.);
#63562=ORIENTED_EDGE('',*,*,#46309,.T.);
#63563=ORIENTED_EDGE('',*,*,#46224,.T.);
#63564=ORIENTED_EDGE('',*,*,#46216,.T.);
#63565=ORIENTED_EDGE('',*,*,#46255,.T.);
#63566=ORIENTED_EDGE('',*,*,#46310,.T.);
#63567=ORIENTED_EDGE('',*,*,#46311,.T.);
#63568=ORIENTED_EDGE('',*,*,#46233,.T.);
#63569=ORIENTED_EDGE('',*,*,#46312,.T.);
#63570=ORIENTED_EDGE('',*,*,#46311,.F.);
#63571=ORIENTED_EDGE('',*,*,#46313,.T.);
#63572=ORIENTED_EDGE('',*,*,#46314,.F.);
#63573=ORIENTED_EDGE('',*,*,#46234,.T.);
#63574=ORIENTED_EDGE('',*,*,#46303,.T.);
#63575=ORIENTED_EDGE('',*,*,#46301,.T.);
#63576=ORIENTED_EDGE('',*,*,#46288,.T.);
#63577=ORIENTED_EDGE('',*,*,#46315,.T.);
#63578=ORIENTED_EDGE('',*,*,#46316,.F.);
#63579=ORIENTED_EDGE('',*,*,#46313,.F.);
#63580=ORIENTED_EDGE('',*,*,#46310,.F.);
#63581=ORIENTED_EDGE('',*,*,#46317,.T.);
#63582=ORIENTED_EDGE('',*,*,#46318,.T.);
#63583=ORIENTED_EDGE('',*,*,#46276,.T.);
#63584=ORIENTED_EDGE('',*,*,#46319,.F.);
#63585=ORIENTED_EDGE('',*,*,#46320,.F.);
#63586=ORIENTED_EDGE('',*,*,#46321,.F.);
#63587=ORIENTED_EDGE('',*,*,#46322,.T.);
#63588=ORIENTED_EDGE('',*,*,#46323,.T.);
#63589=ORIENTED_EDGE('',*,*,#46304,.T.);
#63590=ORIENTED_EDGE('',*,*,#46221,.T.);
#63591=ORIENTED_EDGE('',*,*,#46235,.T.);
#63592=ORIENTED_EDGE('',*,*,#46314,.T.);
#63593=ORIENTED_EDGE('',*,*,#46316,.T.);
#63594=ORIENTED_EDGE('',*,*,#46324,.T.);
#63595=ORIENTED_EDGE('',*,*,#46312,.F.);
#63596=ORIENTED_EDGE('',*,*,#46232,.F.);
#63597=ORIENTED_EDGE('',*,*,#46325,.F.);
#63598=ORIENTED_EDGE('',*,*,#46317,.F.);
#63599=ORIENTED_EDGE('',*,*,#46326,.F.);
#63600=ORIENTED_EDGE('',*,*,#46277,.F.);
#63601=ORIENTED_EDGE('',*,*,#46318,.F.);
#63602=ORIENTED_EDGE('',*,*,#46325,.T.);
#63603=ORIENTED_EDGE('',*,*,#46231,.F.);
#63604=ORIENTED_EDGE('',*,*,#46283,.F.);
#63605=ORIENTED_EDGE('',*,*,#46326,.T.);
#63606=ORIENTED_EDGE('',*,*,#46282,.F.);
#63607=ORIENTED_EDGE('',*,*,#46327,.F.);
#63608=ORIENTED_EDGE('',*,*,#46328,.T.);
#63609=ORIENTED_EDGE('',*,*,#46329,.T.);
#63610=ORIENTED_EDGE('',*,*,#46278,.F.);
#63611=ORIENTED_EDGE('',*,*,#46330,.T.);
#63612=ORIENTED_EDGE('',*,*,#46290,.T.);
#63613=ORIENTED_EDGE('',*,*,#46331,.T.);
#63614=ORIENTED_EDGE('',*,*,#46332,.T.);
#63615=ORIENTED_EDGE('',*,*,#46333,.T.);
#63616=ORIENTED_EDGE('',*,*,#46291,.T.);
#63617=ORIENTED_EDGE('',*,*,#46330,.F.);
#63618=ORIENTED_EDGE('',*,*,#46334,.T.);
#63619=ORIENTED_EDGE('',*,*,#46335,.T.);
#63620=ORIENTED_EDGE('',*,*,#46292,.T.);
#63621=ORIENTED_EDGE('',*,*,#46333,.F.);
#63622=ORIENTED_EDGE('',*,*,#46336,.T.);
#63623=ORIENTED_EDGE('',*,*,#46331,.F.);
#63624=ORIENTED_EDGE('',*,*,#46293,.T.);
#63625=ORIENTED_EDGE('',*,*,#46335,.F.);
#63626=ORIENTED_EDGE('',*,*,#46337,.T.);
#63627=ORIENTED_EDGE('',*,*,#46334,.F.);
#63628=ORIENTED_EDGE('',*,*,#46338,.T.);
#63629=ORIENTED_EDGE('',*,*,#46339,.T.);
#63630=ORIENTED_EDGE('',*,*,#46340,.F.);
#63631=ORIENTED_EDGE('',*,*,#46332,.F.);
#63632=ORIENTED_EDGE('',*,*,#46341,.T.);
#63633=ORIENTED_EDGE('',*,*,#46342,.T.);
#63634=ORIENTED_EDGE('',*,*,#46338,.F.);
#63635=ORIENTED_EDGE('',*,*,#46337,.F.);
#63636=ORIENTED_EDGE('',*,*,#46343,.T.);
#63637=ORIENTED_EDGE('',*,*,#46344,.T.);
#63638=ORIENTED_EDGE('',*,*,#46341,.F.);
#63639=ORIENTED_EDGE('',*,*,#46336,.F.);
#63640=ORIENTED_EDGE('',*,*,#46340,.T.);
#63641=ORIENTED_EDGE('',*,*,#46345,.T.);
#63642=ORIENTED_EDGE('',*,*,#46343,.F.);
#63643=ORIENTED_EDGE('',*,*,#46342,.F.);
#63644=ORIENTED_EDGE('',*,*,#46344,.F.);
#63645=ORIENTED_EDGE('',*,*,#46345,.F.);
#63646=ORIENTED_EDGE('',*,*,#46339,.F.);
#63647=ORIENTED_EDGE('',*,*,#46328,.F.);
#63648=ORIENTED_EDGE('',*,*,#46346,.F.);
#63649=ORIENTED_EDGE('',*,*,#46347,.F.);
#63650=ORIENTED_EDGE('',*,*,#46348,.F.);
#63651=ORIENTED_EDGE('',*,*,#46346,.T.);
#63652=ORIENTED_EDGE('',*,*,#46327,.T.);
#63653=ORIENTED_EDGE('',*,*,#46281,.F.);
#63654=ORIENTED_EDGE('',*,*,#46349,.F.);
#63655=ORIENTED_EDGE('',*,*,#46348,.T.);
#63656=ORIENTED_EDGE('',*,*,#46350,.T.);
#63657=ORIENTED_EDGE('',*,*,#46279,.F.);
#63658=ORIENTED_EDGE('',*,*,#46329,.F.);
#63659=ORIENTED_EDGE('',*,*,#46347,.T.);
#63660=ORIENTED_EDGE('',*,*,#46349,.T.);
#63661=ORIENTED_EDGE('',*,*,#46280,.F.);
#63662=ORIENTED_EDGE('',*,*,#46350,.F.);
#63663=ORIENTED_EDGE('',*,*,#46295,.F.);
#63664=ORIENTED_EDGE('',*,*,#46228,.T.);
#63665=ORIENTED_EDGE('',*,*,#46351,.T.);
#63666=ORIENTED_EDGE('',*,*,#46352,.F.);
#63667=ORIENTED_EDGE('',*,*,#46353,.F.);
#63668=ORIENTED_EDGE('',*,*,#46354,.F.);
#63669=ORIENTED_EDGE('',*,*,#46355,.F.);
#63670=ORIENTED_EDGE('',*,*,#46320,.T.);
#63671=ORIENTED_EDGE('',*,*,#46356,.T.);
#63672=ORIENTED_EDGE('',*,*,#46357,.F.);
#63673=ORIENTED_EDGE('',*,*,#46358,.F.);
#63674=ORIENTED_EDGE('',*,*,#46359,.F.);
#63675=ORIENTED_EDGE('',*,*,#46360,.T.);
#63676=ORIENTED_EDGE('',*,*,#46361,.T.);
#63677=ORIENTED_EDGE('',*,*,#46353,.T.);
#63678=ORIENTED_EDGE('',*,*,#46362,.T.);
#63679=ORIENTED_EDGE('',*,*,#46363,.T.);
#63680=ORIENTED_EDGE('',*,*,#46358,.T.);
#63681=ORIENTED_EDGE('',*,*,#46364,.T.);
#63682=ORIENTED_EDGE('',*,*,#46365,.T.);
#63683=ORIENTED_EDGE('',*,*,#46366,.T.);
#63684=ORIENTED_EDGE('',*,*,#46367,.T.);
#63685=ORIENTED_EDGE('',*,*,#46368,.T.);
#63686=ORIENTED_EDGE('',*,*,#46369,.F.);
#63687=ORIENTED_EDGE('',*,*,#46370,.T.);
#63688=ORIENTED_EDGE('',*,*,#46247,.T.);
#63689=ORIENTED_EDGE('',*,*,#46371,.T.);
#63690=ORIENTED_EDGE('',*,*,#46372,.F.);
#63691=ORIENTED_EDGE('',*,*,#46373,.T.);
#63692=ORIENTED_EDGE('',*,*,#46266,.T.);
#63693=ORIENTED_EDGE('',*,*,#46374,.T.);
#63694=ORIENTED_EDGE('',*,*,#46375,.T.);
#63695=ORIENTED_EDGE('',*,*,#46372,.T.);
#63696=ORIENTED_EDGE('',*,*,#46376,.T.);
#63697=ORIENTED_EDGE('',*,*,#46377,.T.);
#63698=ORIENTED_EDGE('',*,*,#46378,.T.);
#63699=ORIENTED_EDGE('',*,*,#46369,.T.);
#63700=ORIENTED_EDGE('',*,*,#46379,.T.);
#63701=ORIENTED_EDGE('',*,*,#46380,.T.);
#63702=ORIENTED_EDGE('',*,*,#46381,.T.);
#63703=ORIENTED_EDGE('',*,*,#46249,.T.);
#63704=ORIENTED_EDGE('',*,*,#46382,.F.);
#63705=ORIENTED_EDGE('',*,*,#46356,.F.);
#63706=ORIENTED_EDGE('',*,*,#46319,.T.);
#63707=ORIENTED_EDGE('',*,*,#46275,.T.);
#63708=ORIENTED_EDGE('',*,*,#46267,.T.);
#63709=ORIENTED_EDGE('',*,*,#46373,.F.);
#63710=ORIENTED_EDGE('',*,*,#46375,.F.);
#63711=ORIENTED_EDGE('',*,*,#46383,.T.);
#63712=ORIENTED_EDGE('',*,*,#46362,.F.);
#63713=ORIENTED_EDGE('',*,*,#46352,.T.);
#63714=ORIENTED_EDGE('',*,*,#46384,.T.);
#63715=ORIENTED_EDGE('',*,*,#46385,.F.);
#63716=ORIENTED_EDGE('',*,*,#46360,.F.);
#63717=ORIENTED_EDGE('',*,*,#46383,.F.);
#63718=ORIENTED_EDGE('',*,*,#46374,.F.);
#63719=ORIENTED_EDGE('',*,*,#46265,.T.);
#63720=ORIENTED_EDGE('',*,*,#46296,.T.);
#63721=ORIENTED_EDGE('',*,*,#46354,.T.);
#63722=ORIENTED_EDGE('',*,*,#46361,.F.);
#63723=ORIENTED_EDGE('',*,*,#46385,.T.);
#63724=ORIENTED_EDGE('',*,*,#46376,.F.);
#63725=ORIENTED_EDGE('',*,*,#46371,.F.);
#63726=ORIENTED_EDGE('',*,*,#46386,.T.);
#63727=ORIENTED_EDGE('',*,*,#46387,.T.);
#63728=ORIENTED_EDGE('',*,*,#46388,.T.);
#63729=ORIENTED_EDGE('',*,*,#46389,.T.);
#63730=ORIENTED_EDGE('',*,*,#46306,.T.);
#63731=ORIENTED_EDGE('',*,*,#46390,.T.);
#63732=ORIENTED_EDGE('',*,*,#46391,.T.);
#63733=ORIENTED_EDGE('',*,*,#46392,.T.);
#63734=ORIENTED_EDGE('',*,*,#46308,.F.);
#63735=ORIENTED_EDGE('',*,*,#46393,.T.);
#63736=ORIENTED_EDGE('',*,*,#46244,.T.);
#63737=ORIENTED_EDGE('',*,*,#46394,.T.);
#63738=ORIENTED_EDGE('',*,*,#46322,.F.);
#63739=ORIENTED_EDGE('',*,*,#46395,.F.);
#63740=ORIENTED_EDGE('',*,*,#46396,.F.);
#63741=ORIENTED_EDGE('',*,*,#46365,.F.);
#63742=ORIENTED_EDGE('',*,*,#46397,.F.);
#63743=ORIENTED_EDGE('',*,*,#46380,.F.);
#63744=ORIENTED_EDGE('',*,*,#46268,.T.);
#63745=ORIENTED_EDGE('',*,*,#46384,.F.);
#63746=ORIENTED_EDGE('',*,*,#46351,.F.);
#63747=ORIENTED_EDGE('',*,*,#46227,.F.);
#63748=ORIENTED_EDGE('',*,*,#46298,.T.);
#63749=ORIENTED_EDGE('',*,*,#46245,.T.);
#63750=ORIENTED_EDGE('',*,*,#46395,.T.);
#63751=ORIENTED_EDGE('',*,*,#46321,.T.);
#63752=ORIENTED_EDGE('',*,*,#46355,.T.);
#63753=ORIENTED_EDGE('',*,*,#46398,.T.);
#63754=ORIENTED_EDGE('',*,*,#46246,.T.);
#63755=ORIENTED_EDGE('',*,*,#46398,.F.);
#63756=ORIENTED_EDGE('',*,*,#46359,.T.);
#63757=ORIENTED_EDGE('',*,*,#46366,.F.);
#63758=ORIENTED_EDGE('',*,*,#46396,.T.);
#63759=ORIENTED_EDGE('',*,*,#46379,.F.);
#63760=ORIENTED_EDGE('',*,*,#46368,.F.);
#63761=ORIENTED_EDGE('',*,*,#46377,.F.);
#63762=ORIENTED_EDGE('',*,*,#46399,.T.);
#63763=ORIENTED_EDGE('',*,*,#46363,.F.);
#63764=ORIENTED_EDGE('',*,*,#46399,.F.);
#63765=ORIENTED_EDGE('',*,*,#46248,.T.);
#63766=ORIENTED_EDGE('',*,*,#46370,.F.);
#63767=ORIENTED_EDGE('',*,*,#46378,.F.);
#63768=ORIENTED_EDGE('',*,*,#46397,.T.);
#63769=ORIENTED_EDGE('',*,*,#46364,.F.);
#63770=ORIENTED_EDGE('',*,*,#46357,.T.);
#63771=ORIENTED_EDGE('',*,*,#46382,.T.);
#63772=ORIENTED_EDGE('',*,*,#46324,.F.);
#63773=ORIENTED_EDGE('',*,*,#46315,.F.);
#63774=ORIENTED_EDGE('',*,*,#46287,.F.);
#63775=ORIENTED_EDGE('',*,*,#46236,.F.);
#63776=ORIENTED_EDGE('',*,*,#46389,.F.);
#63777=ORIENTED_EDGE('',*,*,#46400,.F.);
#63778=ORIENTED_EDGE('',*,*,#46393,.F.);
#63779=ORIENTED_EDGE('',*,*,#46307,.T.);
#63780=ORIENTED_EDGE('',*,*,#46387,.F.);
#63781=ORIENTED_EDGE('',*,*,#46401,.T.);
#63782=ORIENTED_EDGE('',*,*,#46391,.F.);
#63783=ORIENTED_EDGE('',*,*,#46401,.F.);
#63784=ORIENTED_EDGE('',*,*,#46367,.F.);
#63785=ORIENTED_EDGE('',*,*,#46402,.T.);
#63786=ORIENTED_EDGE('',*,*,#46381,.F.);
#63787=ORIENTED_EDGE('',*,*,#46402,.F.);
#63788=ORIENTED_EDGE('',*,*,#46386,.F.);
#63789=ORIENTED_EDGE('',*,*,#46403,.T.);
#63790=ORIENTED_EDGE('',*,*,#46305,.T.);
#63791=ORIENTED_EDGE('',*,*,#46323,.F.);
#63792=ORIENTED_EDGE('',*,*,#46394,.F.);
#63793=ORIENTED_EDGE('',*,*,#46243,.T.);
#63794=ORIENTED_EDGE('',*,*,#46300,.F.);
#63795=ORIENTED_EDGE('',*,*,#46270,.T.);
#63796=ORIENTED_EDGE('',*,*,#46299,.F.);
#63797=ORIENTED_EDGE('',*,*,#46225,.F.);
#63798=ORIENTED_EDGE('',*,*,#46309,.F.);
#63799=ORIENTED_EDGE('',*,*,#46404,.T.);
#63800=ORIENTED_EDGE('',*,*,#46390,.F.);
#63801=ORIENTED_EDGE('',*,*,#46404,.F.);
#63802=ORIENTED_EDGE('',*,*,#46392,.F.);
#63803=ORIENTED_EDGE('',*,*,#46400,.T.);
#63804=ORIENTED_EDGE('',*,*,#46388,.F.);
#63805=ORIENTED_EDGE('',*,*,#46403,.F.);
#87504=CYLINDRICAL_SURFACE('',#97132,8.);
#87505=CYLINDRICAL_SURFACE('',#97133,4.);
#87506=CYLINDRICAL_SURFACE('',#97135,10.25);
#87507=CYLINDRICAL_SURFACE('',#97141,1.);
#87508=CYLINDRICAL_SURFACE('',#97150,1.);
#87509=CYLINDRICAL_SURFACE('',#97154,1.7);
#87510=CYLINDRICAL_SURFACE('',#97163,3.2);
#87511=CYLINDRICAL_SURFACE('',#97166,3.2);
#87512=CYLINDRICAL_SURFACE('',#97172,1.7);
#87513=CYLINDRICAL_SURFACE('',#97197,8.);
#87514=CYLINDRICAL_SURFACE('',#97198,3.);
#87515=CYLINDRICAL_SURFACE('',#97200,3.);
#87516=CYLINDRICAL_SURFACE('',#97213,5.);
#87517=CYLINDRICAL_SURFACE('',#97214,5.);
#87518=CYLINDRICAL_SURFACE('',#97215,3.);
#87519=CYLINDRICAL_SURFACE('',#97216,1.5);
#87520=CYLINDRICAL_SURFACE('',#97217,3.);
#87521=CYLINDRICAL_SURFACE('',#97220,1.6);
#87522=CYLINDRICAL_SURFACE('',#97221,1.5);
#87523=CYLINDRICAL_SURFACE('',#97222,4.);
#89828=ADVANCED_FACE('',(#7364),#5547,.F.);
#89829=ADVANCED_FACE('',(#7365),#5548,.F.);
#89830=ADVANCED_FACE('',(#7366),#5549,.F.);
#89831=ADVANCED_FACE('',(#7367),#5550,.F.);
#89832=ADVANCED_FACE('',(#7368),#5551,.T.);
#89833=ADVANCED_FACE('',(#7369),#5552,.T.);
#89834=ADVANCED_FACE('',(#7370),#5553,.T.);
#89835=ADVANCED_FACE('',(#7371),#5554,.T.);
#89836=ADVANCED_FACE('',(#7372,#5162),#5555,.T.);
#89837=ADVANCED_FACE('',(#7373),#5556,.F.);
#89838=ADVANCED_FACE('',(#7374),#5557,.F.);
#89839=ADVANCED_FACE('',(#7375),#87504,.F.);
#89840=ADVANCED_FACE('',(#7376),#87505,.T.);
#89841=ADVANCED_FACE('',(#7377),#5558,.T.);
#89842=ADVANCED_FACE('',(#7378),#87506,.F.);
#89843=ADVANCED_FACE('',(#7379),#5559,.F.);
#89844=ADVANCED_FACE('',(#7380),#5560,.F.);
#89845=ADVANCED_FACE('',(#7381),#5561,.F.);
#89846=ADVANCED_FACE('',(#7382),#5562,.T.);
#89847=ADVANCED_FACE('',(#7383),#87507,.T.);
#89848=ADVANCED_FACE('',(#7384),#5563,.T.);
#89849=ADVANCED_FACE('',(#7385),#5564,.F.);
#89850=ADVANCED_FACE('',(#7386),#87508,.T.);
#89851=ADVANCED_FACE('',(#7387),#5565,.F.);
#89852=ADVANCED_FACE('',(#7388),#5566,.F.);
#89853=ADVANCED_FACE('',(#7389),#87509,.F.);
#89854=ADVANCED_FACE('',(#7390),#4702,.F.);
#89855=ADVANCED_FACE('',(#7391),#5567,.T.);
#89856=ADVANCED_FACE('',(#7392),#4703,.F.);
#89857=ADVANCED_FACE('',(#7393),#5568,.T.);
#89858=ADVANCED_FACE('',(#7394),#5569,.F.);
#89859=ADVANCED_FACE('',(#7395),#87510,.F.);
#89860=ADVANCED_FACE('',(#7396),#5570,.F.);
#89861=ADVANCED_FACE('',(#7397),#87511,.F.);
#89862=ADVANCED_FACE('',(#7398,#5163),#5571,.T.);
#89863=ADVANCED_FACE('',(#7399),#5572,.F.);
#89864=ADVANCED_FACE('',(#7400),#5573,.F.);
#89865=ADVANCED_FACE('',(#7401),#87512,.F.);
#89866=ADVANCED_FACE('',(#7402),#4704,.T.);
#89867=ADVANCED_FACE('',(#7403),#4705,.T.);
#89868=ADVANCED_FACE('',(#7404,#5164),#5574,.T.);
#89869=ADVANCED_FACE('',(#7405,#5165),#5575,.T.);
#89870=ADVANCED_FACE('',(#7406),#4706,.T.);
#89871=ADVANCED_FACE('',(#7407),#4707,.T.);
#89872=ADVANCED_FACE('',(#7408,#5166),#5576,.T.);
#89873=ADVANCED_FACE('',(#7409,#5167),#5577,.T.);
#89874=ADVANCED_FACE('',(#7410),#87513,.F.);
#89875=ADVANCED_FACE('',(#7411),#87514,.T.);
#89876=ADVANCED_FACE('',(#7412),#5578,.T.);
#89877=ADVANCED_FACE('',(#7413),#87515,.T.);
#89878=ADVANCED_FACE('',(#7414,#5168),#5579,.T.);
#89879=ADVANCED_FACE('',(#7415),#5580,.F.);
#89880=ADVANCED_FACE('',(#7416,#5169),#5581,.T.);
#89881=ADVANCED_FACE('',(#7417),#5582,.F.);
#89882=ADVANCED_FACE('',(#7418),#5583,.T.);
#89883=ADVANCED_FACE('',(#7419),#5584,.T.);
#89884=ADVANCED_FACE('',(#7420),#87516,.F.);
#89885=ADVANCED_FACE('',(#7421),#87517,.F.);
#89886=ADVANCED_FACE('',(#7422),#87518,.T.);
#89887=ADVANCED_FACE('',(#7423),#87519,.F.);
#89888=ADVANCED_FACE('',(#7424),#87520,.T.);
#89889=ADVANCED_FACE('',(#7425),#5585,.T.);
#89890=ADVANCED_FACE('',(#7426),#5586,.T.);
#89891=ADVANCED_FACE('',(#7427),#87521,.F.);
#89892=ADVANCED_FACE('',(#7428),#87522,.F.);
#89893=ADVANCED_FACE('',(#7429),#87523,.T.);
#94629=CLOSED_SHELL('',(#89828,#89829,#89830,#89831,#89832,#89833,#89834,
#89835,#89836,#89837,#89838,#89839,#89840,#89841,#89842,#89843,#89844,#89845,
#89846,#89847,#89848,#89849,#89850,#89851,#89852,#89853,#89854,#89855,#89856,
#89857,#89858,#89859,#89860,#89861,#89862,#89863,#89864,#89865,#89866,#89867,
#89868,#89869,#89870,#89871,#89872,#89873,#89874,#89875,#89876,#89877,#89878,
#89879,#89880,#89881,#89882,#89883,#89884,#89885,#89886,#89887,#89888,#89889,
#89890,#89891,#89892,#89893));
#97093=AXIS2_PLACEMENT_3D('',#145398,#111075,#111076);
#97094=AXIS2_PLACEMENT_3D('',#145399,#111077,#111078);
#97095=AXIS2_PLACEMENT_3D('',#145408,#111083,#111084);
#97096=AXIS2_PLACEMENT_3D('',#145417,#111089,#111090);
#97097=AXIS2_PLACEMENT_3D('',#145423,#111093,#111094);
#97098=AXIS2_PLACEMENT_3D('',#145427,#111096,#111097);
#97099=AXIS2_PLACEMENT_3D('',#145429,#111098,#111099);
#97100=AXIS2_PLACEMENT_3D('',#145431,#111100,#111101);
#97101=AXIS2_PLACEMENT_3D('',#145439,#111105,#111106);
#97102=AXIS2_PLACEMENT_3D('',#145443,#111108,#111109);
#97103=AXIS2_PLACEMENT_3D('',#145449,#111113,#111114);
#97104=AXIS2_PLACEMENT_3D('',#145455,#111117,#111118);
#97105=AXIS2_PLACEMENT_3D('',#145457,#111119,#111120);
#97106=AXIS2_PLACEMENT_3D('',#145459,#111121,#111122);
#97107=AXIS2_PLACEMENT_3D('',#145463,#111124,#111125);
#97108=AXIS2_PLACEMENT_3D('',#145465,#111126,#111127);
#97109=AXIS2_PLACEMENT_3D('',#145467,#111128,#111129);
#97110=AXIS2_PLACEMENT_3D('',#145469,#111130,#111131);
#97111=AXIS2_PLACEMENT_3D('',#145471,#111132,#111133);
#97112=AXIS2_PLACEMENT_3D('',#145481,#111139,#111140);
#97113=AXIS2_PLACEMENT_3D('',#145486,#111144,#111145);
#97114=AXIS2_PLACEMENT_3D('',#145500,#111152,#111153);
#97115=AXIS2_PLACEMENT_3D('',#145502,#111154,#111155);
#97116=AXIS2_PLACEMENT_3D('',#145504,#111156,#111157);
#97117=AXIS2_PLACEMENT_3D('',#145506,#111158,#111159);
#97118=AXIS2_PLACEMENT_3D('',#145508,#111160,#111161);
#97119=AXIS2_PLACEMENT_3D('',#145512,#111163,#111164);
#97120=AXIS2_PLACEMENT_3D('',#145514,#111165,#111166);
#97121=AXIS2_PLACEMENT_3D('',#145515,#111167,#111168);
#97122=AXIS2_PLACEMENT_3D('',#145516,#111169,#111170);
#97123=AXIS2_PLACEMENT_3D('',#145519,#111173,#111174);
#97124=AXIS2_PLACEMENT_3D('',#145527,#111178,#111179);
#97125=AXIS2_PLACEMENT_3D('',#145531,#111181,#111182);
#97126=AXIS2_PLACEMENT_3D('',#145535,#111184,#111185);
#97127=AXIS2_PLACEMENT_3D('',#145538,#111188,#111189);
#97128=AXIS2_PLACEMENT_3D('',#145548,#111195,#111196);
#97129=AXIS2_PLACEMENT_3D('',#145552,#111198,#111199);
#97130=AXIS2_PLACEMENT_3D('',#145554,#111201,#111202);
#97131=AXIS2_PLACEMENT_3D('',#145556,#111204,#111205);
#97132=AXIS2_PLACEMENT_3D('',#145557,#111206,#111207);
#97133=AXIS2_PLACEMENT_3D('',#145566,#111209,#111210);
#97134=AXIS2_PLACEMENT_3D('',#145568,#111212,#111213);
#97135=AXIS2_PLACEMENT_3D('',#145571,#111216,#111217);
#97136=AXIS2_PLACEMENT_3D('',#145573,#111219,#111220);
#97137=AXIS2_PLACEMENT_3D('',#145577,#111223,#111224);
#97138=AXIS2_PLACEMENT_3D('',#145579,#111226,#111227);
#97139=AXIS2_PLACEMENT_3D('',#145580,#111228,#111229);
#97140=AXIS2_PLACEMENT_3D('',#145591,#111235,#111236);
#97141=AXIS2_PLACEMENT_3D('',#145592,#111237,#111238);
#97142=AXIS2_PLACEMENT_3D('',#145595,#111239,#111240);
#97143=AXIS2_PLACEMENT_3D('',#145598,#111243,#111244);
#97144=AXIS2_PLACEMENT_3D('',#145602,#111247,#111248);
#97145=AXIS2_PLACEMENT_3D('',#145605,#111250,#111251);
#97146=AXIS2_PLACEMENT_3D('',#145610,#111254,#111255);
#97147=AXIS2_PLACEMENT_3D('',#145612,#111256,#111257);
#97148=AXIS2_PLACEMENT_3D('',#145614,#111258,#111259);
#97149=AXIS2_PLACEMENT_3D('',#145617,#111261,#111262);
#97150=AXIS2_PLACEMENT_3D('',#145618,#111263,#111264);
#97151=AXIS2_PLACEMENT_3D('',#145620,#111266,#111267);
#97152=AXIS2_PLACEMENT_3D('',#145622,#111269,#111270);
#97153=AXIS2_PLACEMENT_3D('',#145623,#111271,#111272);
#97154=AXIS2_PLACEMENT_3D('',#145624,#111273,#111274);
#97155=AXIS2_PLACEMENT_3D('',#145628,#111276,#111277);
#97156=AXIS2_PLACEMENT_3D('',#145630,#111279,#111280);
#97157=AXIS2_PLACEMENT_3D('',#145635,#111283,#111284);
#97158=AXIS2_PLACEMENT_3D('',#145636,#111285,#111286);
#97159=AXIS2_PLACEMENT_3D('',#145640,#111289,#111290);
#97160=AXIS2_PLACEMENT_3D('',#145643,#111292,#111293);
#97161=AXIS2_PLACEMENT_3D('',#145644,#111294,#111295);
#97162=AXIS2_PLACEMENT_3D('',#145646,#111297,#111298);
#97163=AXIS2_PLACEMENT_3D('',#145652,#111302,#111303);
#97164=AXIS2_PLACEMENT_3D('',#145655,#111305,#111306);
#97165=AXIS2_PLACEMENT_3D('',#145656,#111307,#111308);
#97166=AXIS2_PLACEMENT_3D('',#145660,#111311,#111312);
#97167=AXIS2_PLACEMENT_3D('',#145661,#111313,#111314);
#97168=AXIS2_PLACEMENT_3D('',#145662,#111315,#111316);
#97169=AXIS2_PLACEMENT_3D('',#145666,#111318,#111319);
#97170=AXIS2_PLACEMENT_3D('',#145668,#111321,#111322);
#97171=AXIS2_PLACEMENT_3D('',#145670,#111324,#111325);
#97172=AXIS2_PLACEMENT_3D('',#145672,#111327,#111328);
#97173=AXIS2_PLACEMENT_3D('',#145673,#111329,#111330);
#97174=AXIS2_PLACEMENT_3D('',#145689,#111331,#111332);
#97175=AXIS2_PLACEMENT_3D('',#145698,#111333,#111334);
#97176=AXIS2_PLACEMENT_3D('',#145723,#111335,#111336);
#97177=AXIS2_PLACEMENT_3D('',#145730,#111337,#111338);
#97178=AXIS2_PLACEMENT_3D('',#145734,#111340,#111341);
#97179=AXIS2_PLACEMENT_3D('',#145735,#111342,#111343);
#97180=AXIS2_PLACEMENT_3D('',#145737,#111344,#111345);
#97181=AXIS2_PLACEMENT_3D('',#145738,#111346,#111347);
#97182=AXIS2_PLACEMENT_3D('',#145740,#111348,#111349);
#97183=AXIS2_PLACEMENT_3D('',#145743,#111351,#111352);
#97184=AXIS2_PLACEMENT_3D('',#145745,#111353,#111354);
#97185=AXIS2_PLACEMENT_3D('',#145746,#111355,#111356);
#97186=AXIS2_PLACEMENT_3D('',#145753,#111357,#111358);
#97187=AXIS2_PLACEMENT_3D('',#145760,#111359,#111360);
#97188=AXIS2_PLACEMENT_3D('',#145769,#111361,#111362);
#97189=AXIS2_PLACEMENT_3D('',#145774,#111363,#111364);
#97190=AXIS2_PLACEMENT_3D('',#145778,#111366,#111367);
#97191=AXIS2_PLACEMENT_3D('',#145779,#111368,#111369);
#97192=AXIS2_PLACEMENT_3D('',#145781,#111370,#111371);
#97193=AXIS2_PLACEMENT_3D('',#145782,#111372,#111373);
#97194=AXIS2_PLACEMENT_3D('',#145784,#111374,#111375);
#97195=AXIS2_PLACEMENT_3D('',#145786,#111376,#111377);
#97196=AXIS2_PLACEMENT_3D('',#145789,#111379,#111380);
#97197=AXIS2_PLACEMENT_3D('',#145790,#111381,#111382);
#97198=AXIS2_PLACEMENT_3D('',#145792,#111384,#111385);
#97199=AXIS2_PLACEMENT_3D('',#145795,#111388,#111389);
#97200=AXIS2_PLACEMENT_3D('',#145797,#111391,#111392);
#97201=AXIS2_PLACEMENT_3D('',#145798,#111393,#111394);
#97202=AXIS2_PLACEMENT_3D('',#145800,#111395,#111396);
#97203=AXIS2_PLACEMENT_3D('',#145802,#111397,#111398);
#97204=AXIS2_PLACEMENT_3D('',#145803,#111399,#111400);
#97205=AXIS2_PLACEMENT_3D('',#145805,#111401,#111402);
#97206=AXIS2_PLACEMENT_3D('',#145807,#111404,#111405);
#97207=AXIS2_PLACEMENT_3D('',#145809,#111406,#111407);
#97208=AXIS2_PLACEMENT_3D('',#145811,#111408,#111409);
#97209=AXIS2_PLACEMENT_3D('',#145812,#111410,#111411);
#97210=AXIS2_PLACEMENT_3D('',#145814,#111412,#111413);
#97211=AXIS2_PLACEMENT_3D('',#145816,#111415,#111416);
#97212=AXIS2_PLACEMENT_3D('',#145819,#111419,#111420);
#97213=AXIS2_PLACEMENT_3D('',#145822,#111423,#111424);
#97214=AXIS2_PLACEMENT_3D('',#145823,#111425,#111426);
#97215=AXIS2_PLACEMENT_3D('',#145825,#111428,#111429);
#97216=AXIS2_PLACEMENT_3D('',#145826,#111430,#111431);
#97217=AXIS2_PLACEMENT_3D('',#145828,#111433,#111434);
#97218=AXIS2_PLACEMENT_3D('',#145829,#111435,#111436);
#97219=AXIS2_PLACEMENT_3D('',#145830,#111437,#111438);
#97220=AXIS2_PLACEMENT_3D('',#145832,#111440,#111441);
#97221=AXIS2_PLACEMENT_3D('',#145834,#111443,#111444);
#97222=AXIS2_PLACEMENT_3D('',#145836,#111446,#111447);
#111075=DIRECTION('axis',(0.,0.,1.));
#111076=DIRECTION('refdir',(1.,0.,0.));
#111077=DIRECTION('center_axis',(-0.707106781186547,8.2927418592453E-17,
-0.707106781186548));
#111078=DIRECTION('ref_axis',(-0.707106781186548,-7.08402960210301E-17,
0.707106781186547));
#111079=DIRECTION('',(-0.707106781186548,-7.04136402448282E-17,0.707106781186547));
#111080=DIRECTION('',(8.39504102067944E-47,-1.,-1.17277080066038E-16));
#111081=DIRECTION('',(0.707106781186548,7.04136402448282E-17,-0.707106781186547));
#111082=DIRECTION('',(0.,1.,1.17277080066038E-16));
#111083=DIRECTION('center_axis',(-0.707106781186547,8.2927418592453E-17,
-0.707106781186548));
#111084=DIRECTION('ref_axis',(-0.707106781186548,-7.08402960210301E-17,
0.707106781186547));
#111085=DIRECTION('',(0.707106781186548,7.04136402448282E-17,-0.707106781186547));
#111086=DIRECTION('',(0.,1.,1.17277080066038E-16));
#111087=DIRECTION('',(-0.707106781186548,-7.04136402448282E-17,0.707106781186547));
#111088=DIRECTION('',(8.39504102067944E-47,-1.,-1.17277080066038E-16));
#111089=DIRECTION('center_axis',(8.40594773455218E-47,-1.,-9.9579925010296E-17));
#111090=DIRECTION('ref_axis',(-1.,-8.46731860157208E-47,6.16297582203915E-33));
#111091=DIRECTION('',(1.55426471955831E-12,9.9579925010296E-17,-1.));
#111092=DIRECTION('',(6.16297582203915E-33,-9.9579925010296E-17,1.));
#111093=DIRECTION('center_axis',(8.40594773455218E-47,-1.,-9.9579925010296E-17));
#111094=DIRECTION('ref_axis',(-1.,-8.46731860157208E-47,6.16297582203915E-33));
#111095=DIRECTION('',(6.16297582203915E-33,-9.9579925010296E-17,1.));
#111096=DIRECTION('center_axis',(-8.40594773455218E-47,1.,9.9579925010296E-17));
#111097=DIRECTION('ref_axis',(0.12,-9.88603496856012E-17,0.992773891679268));
#111098=DIRECTION('center_axis',(-8.40594773455218E-47,1.,9.9579925010296E-17));
#111099=DIRECTION('ref_axis',(1.,8.46731860157208E-47,-6.16297582203915E-33));
#111100=DIRECTION('center_axis',(-8.40594773455218E-47,1.,9.9579925010296E-17));
#111101=DIRECTION('ref_axis',(0.0625000000000002,9.93852426637541E-17,-0.998044963916957));
#111102=DIRECTION('',(6.16297582203915E-33,-9.9579925010296E-17,1.));
#111103=DIRECTION('',(0.707106781186551,-7.04136402448278E-17,0.707106781186544));
#111104=DIRECTION('',(-8.88178419700125E-16,-9.9579925010296E-17,1.));
#111105=DIRECTION('center_axis',(8.40594773455218E-47,-1.,-9.9579925010296E-17));
#111106=DIRECTION('ref_axis',(-0.923879532511287,-3.81075874975982E-17,
0.382683432365088));
#111107=DIRECTION('',(-0.707106781186546,7.04136402448283E-17,-0.707106781186548));
#111108=DIRECTION('center_axis',(8.40594773455218E-47,-1.,-9.9579925010296E-17));
#111109=DIRECTION('ref_axis',(-0.38268343236509,-9.19998545660213E-17,0.923879532511287));
#111110=DIRECTION('',(1.,8.46731860157208E-47,-6.16297582203915E-33));
#111111=DIRECTION('',(6.16297582203915E-33,-9.9579925010296E-17,1.));
#111112=DIRECTION('',(-0.707106781186547,7.04136402448282E-17,-0.707106781186548));
#111113=DIRECTION('center_axis',(8.40594773455218E-47,-1.,-9.9579925010296E-17));
#111114=DIRECTION('ref_axis',(-1.,-8.46731860157208E-47,6.16297582203915E-33));
#111115=DIRECTION('',(1.55426471955831E-12,9.9579925010296E-17,-1.));
#111116=DIRECTION('',(-0.899167304897951,-4.35766755619441E-17,0.437605024882661));
#111117=DIRECTION('center_axis',(6.9388939039071E-18,1.,9.95799250102971E-17));
#111118=DIRECTION('ref_axis',(0.999999893270433,-6.98490071851115E-18,0.000462016367098532));
#111119=DIRECTION('center_axis',(8.40594773455218E-47,-1.,-9.9579925010296E-17));
#111120=DIRECTION('ref_axis',(-1.,-8.46731860157208E-47,6.16297582203915E-33));
#111121=DIRECTION('center_axis',(6.9388939039071E-18,1.,9.95799250102971E-17));
#111122=DIRECTION('ref_axis',(0.999999893270433,-6.98490071851115E-18,0.000462016367098532));
#111123=DIRECTION('',(-6.16297582203915E-33,9.95799250102971E-17,-1.));
#111124=DIRECTION('center_axis',(-8.40594773455218E-47,1.,9.9579925010296E-17));
#111125=DIRECTION('ref_axis',(0.12,-9.88603496856012E-17,0.992773891679268));
#111126=DIRECTION('center_axis',(8.40594773455218E-47,-1.,-9.9579925010296E-17));
#111127=DIRECTION('ref_axis',(-0.85146931829632,5.22201532254593E-17,-0.524404424085075));
#111128=DIRECTION('center_axis',(-8.40594773455218E-47,1.,9.9579925010296E-17));
#111129=DIRECTION('ref_axis',(1.,8.46731860157208E-47,-6.16297582203915E-33));
#111130=DIRECTION('center_axis',(8.40594773455218E-47,-1.,-9.9579925010296E-17));
#111131=DIRECTION('ref_axis',(-0.811844140885989,-5.81421498601493E-17,
0.583874208121142));
#111132=DIRECTION('center_axis',(6.9388939039071E-18,1.,9.95799250102971E-17));
#111133=DIRECTION('ref_axis',(0.0625000000000002,9.93852426637541E-17,-0.998044963916957));
#111134=DIRECTION('',(6.16297582203915E-33,-9.9579925010296E-17,1.));
#111135=DIRECTION('',(0.707106781186547,7.04136402448282E-17,-0.707106781186548));
#111136=DIRECTION('',(1.,0.,0.));
#111137=DIRECTION('',(6.16297582203915E-33,-1.14933685332317E-16,1.));
#111138=DIRECTION('',(0.707106781186547,-8.12703882852425E-17,0.707106781186548));
#111139=DIRECTION('center_axis',(0.437605024882661,-8.53227559733209E-17,
0.899167304897951));
#111140=DIRECTION('ref_axis',(0.899167304897951,3.73374490313955E-17,-0.437605024882661));
#111141=DIRECTION('',(8.40384663814132E-47,-1.,-1.02989148852055E-16));
#111142=DIRECTION('',(-0.899167304897951,-4.35766755619441E-17,0.437605024882661));
#111143=DIRECTION('',(0.,-1.,0.));
#111144=DIRECTION('center_axis',(8.40594773455218E-47,-1.,-9.9579925010296E-17));
#111145=DIRECTION('ref_axis',(-1.,-8.46731860157208E-47,6.16297582203915E-33));
#111146=DIRECTION('',(-1.55426471955831E-12,-9.9579925010296E-17,1.));
#111147=DIRECTION('',(-0.707106781186547,8.12703882852425E-17,-0.707106781186548));
#111148=DIRECTION('',(-6.16297582203915E-33,1.14933685332317E-16,-1.));
#111149=DIRECTION('',(-1.,1.15873958031682E-16,1.83750175990223E-19));
#111150=DIRECTION('',(-0.707106781186547,-7.04136402448282E-17,0.707106781186548));
#111151=DIRECTION('',(-6.16297582203915E-33,9.9579925010296E-17,-1.));
#111152=DIRECTION('center_axis',(-6.9388939039071E-18,-1.,-9.95799250102971E-17));
#111153=DIRECTION('ref_axis',(0.0625000000000002,9.93852426637541E-17,-0.998044963916957));
#111154=DIRECTION('center_axis',(-8.40594773455218E-47,1.,9.9579925010296E-17));
#111155=DIRECTION('ref_axis',(-0.811844140885989,-5.81421498601493E-17,
0.583874208121142));
#111156=DIRECTION('center_axis',(8.40594773455218E-47,-1.,-9.9579925010296E-17));
#111157=DIRECTION('ref_axis',(1.,8.46731860157208E-47,-6.16297582203915E-33));
#111158=DIRECTION('center_axis',(-8.40594773455218E-47,1.,9.9579925010296E-17));
#111159=DIRECTION('ref_axis',(-0.85146931829632,5.22201532254593E-17,-0.524404424085075));
#111160=DIRECTION('center_axis',(8.40594773455218E-47,-1.,-9.9579925010296E-17));
#111161=DIRECTION('ref_axis',(0.12,-9.88603496856012E-17,0.992773891679268));
#111162=DIRECTION('',(6.16297582203915E-33,-9.95799250102971E-17,1.));
#111163=DIRECTION('center_axis',(-6.9388939039071E-18,-1.,-9.95799250102971E-17));
#111164=DIRECTION('ref_axis',(0.999999893270433,-6.98490071851115E-18,0.000462016367098532));
#111165=DIRECTION('center_axis',(-8.40594773455218E-47,1.,9.9579925010296E-17));
#111166=DIRECTION('ref_axis',(-1.,-8.46731860157208E-47,6.16297582203915E-33));
#111167=DIRECTION('center_axis',(-6.9388939039071E-18,-1.,-9.95799250102971E-17));
#111168=DIRECTION('ref_axis',(0.999999893270433,-6.98490071851115E-18,0.000462016367098532));
#111169=DIRECTION('center_axis',(-0.707106781186548,-5.98729840163861E-47,
-0.707106781186547));
#111170=DIRECTION('ref_axis',(-0.707106781186547,0.,0.707106781186548));
#111171=DIRECTION('',(8.46731860157208E-47,-1.,-1.55587128320416E-65));
#111172=DIRECTION('',(-8.46731860157208E-47,1.,1.55587128320416E-65));
#111173=DIRECTION('center_axis',(-1.,-8.46731860157208E-47,6.16297582203915E-33));
#111174=DIRECTION('ref_axis',(-6.16297582203915E-33,9.9579925010296E-17,
-1.));
#111175=DIRECTION('',(-8.40594773455218E-47,1.,9.9579925010296E-17));
#111176=DIRECTION('',(6.16297582203915E-33,-9.9579925010296E-17,1.));
#111177=DIRECTION('',(-8.40594773455218E-47,1.,9.9579925010296E-17));
#111178=DIRECTION('center_axis',(1.,8.46731860157208E-47,-6.16297582203915E-33));
#111179=DIRECTION('ref_axis',(-8.40594773455218E-47,1.,9.9579925010296E-17));
#111180=DIRECTION('',(-6.16297582203915E-33,9.9579925010296E-17,-1.));
#111181=DIRECTION('center_axis',(1.,8.46731860157208E-47,-6.16297582203915E-33));
#111182=DIRECTION('ref_axis',(8.40594773455218E-47,-1.,-9.9579925010296E-17));
#111183=DIRECTION('',(6.16297582203915E-33,-9.9579925010296E-17,1.));
#111184=DIRECTION('center_axis',(1.,8.46731860157208E-47,-6.16297582203915E-33));
#111185=DIRECTION('ref_axis',(-8.40594773455218E-47,1.,9.9579925010296E-17));
#111186=DIRECTION('',(-8.40594773455218E-47,1.,9.9579925010296E-17));
#111187=DIRECTION('',(-8.40594773455218E-47,1.,9.9579925010296E-17));
#111188=DIRECTION('center_axis',(1.,8.46731860157208E-47,-6.16297582203915E-33));
#111189=DIRECTION('ref_axis',(6.16297582203915E-33,-9.9579925010296E-17,
1.));
#111190=DIRECTION('',(-8.46731860157208E-47,1.,0.));
#111191=DIRECTION('',(-8.13081314298998E-47,1.,5.46011323586143E-16));
#111192=DIRECTION('',(-8.40594773455218E-47,1.,9.9579925010296E-17));
#111193=DIRECTION('',(-6.16297582203915E-33,9.9579925010296E-17,-1.));
#111194=DIRECTION('',(-8.13081314298998E-47,1.,5.46011323586143E-16));
#111195=DIRECTION('center_axis',(1.,8.46731860157208E-47,-6.16297582203915E-33));
#111196=DIRECTION('ref_axis',(-8.40594773455218E-47,1.,9.9579925010296E-17));
#111197=DIRECTION('',(6.16297582203915E-33,-9.9579925010296E-17,1.));
#111198=DIRECTION('center_axis',(1.,8.46731860157208E-47,-6.16297582203915E-33));
#111199=DIRECTION('ref_axis',(8.40594773455218E-47,-1.,-9.9579925010296E-17));
#111200=DIRECTION('',(-6.16297582203915E-33,9.9579925010296E-17,-1.));
#111201=DIRECTION('center_axis',(-0.707106781186548,-3.86088309512404E-16,
0.707106781186547));
#111202=DIRECTION('ref_axis',(0.707106781186547,-4.12156156691976E-16,0.707106781186548));
#111203=DIRECTION('',(1.26831058763807E-43,1.,5.46011323586143E-16));
#111204=DIRECTION('center_axis',(1.83750175990223E-19,0.,1.));
#111205=DIRECTION('ref_axis',(-1.,1.15873958031682E-16,1.83750175990223E-19));
#111206=DIRECTION('center_axis',(8.40594773455218E-47,-1.,-9.9579925010296E-17));
#111207=DIRECTION('ref_axis',(0.0625000000000002,9.93852426637541E-17,-0.998044963916957));
#111208=DIRECTION('',(-8.40594773455218E-47,1.,9.9579925010296E-17));
#111209=DIRECTION('center_axis',(0.,-1.,0.));
#111210=DIRECTION('ref_axis',(0.999999893270433,0.,0.000462016367098532));
#111211=DIRECTION('',(0.,1.,0.));
#111212=DIRECTION('center_axis',(-1.,-8.46731860157208E-47,6.16297582203915E-33));
#111213=DIRECTION('ref_axis',(-6.16297582203915E-33,9.9579925010296E-17,
-1.));
#111214=DIRECTION('',(8.40594773455218E-47,-1.,-9.9579925010296E-17));
#111215=DIRECTION('',(8.40594773455218E-47,-1.,-9.9579925010296E-17));
#111216=DIRECTION('center_axis',(8.40594773455218E-47,-1.,-9.9579925010296E-17));
#111217=DIRECTION('ref_axis',(-1.,-8.46731860157208E-47,6.16297582203915E-33));
#111218=DIRECTION('',(0.,-1.,0.));
#111219=DIRECTION('center_axis',(-0.707106781186548,-3.86088309512404E-16,
0.707106781186547));
#111220=DIRECTION('ref_axis',(0.707106781186547,-4.12156156691976E-16,0.707106781186548));
#111221=DIRECTION('',(0.707106781186547,-7.04136402448282E-17,0.707106781186548));
#111222=DIRECTION('',(1.26831058763807E-43,1.,5.46011323586143E-16));
#111223=DIRECTION('center_axis',(-1.,-1.02762453955456E-27,1.88205719398865E-12));
#111224=DIRECTION('ref_axis',(1.88205719398865E-12,-5.82876826609362E-16,
1.));
#111225=DIRECTION('',(-1.55426471955831E-12,-9.9579925010296E-17,1.));
#111226=DIRECTION('center_axis',(-1.,-1.02762453955456E-27,1.88205719398865E-12));
#111227=DIRECTION('ref_axis',(1.88205719398865E-12,-5.82876826609362E-16,
1.));
#111228=DIRECTION('center_axis',(1.,8.46731860157208E-47,-6.16297582203915E-33));
#111229=DIRECTION('ref_axis',(6.16297582203915E-33,-9.9579925010296E-17,
1.));
#111230=DIRECTION('',(-6.16297582203915E-33,9.9579925010296E-17,-1.));
#111231=DIRECTION('',(-6.16297582203915E-33,9.9579925010296E-17,-1.));
#111232=DIRECTION('',(-6.16297582203915E-33,9.9579925010296E-17,-1.));
#111233=DIRECTION('',(8.40594773455218E-47,-1.,-9.9579925010296E-17));
#111234=DIRECTION('',(6.16297582203915E-33,-9.9579925010296E-17,1.));
#111235=DIRECTION('center_axis',(8.40594773455218E-47,-1.,-9.9579925010296E-17));
#111236=DIRECTION('ref_axis',(-1.,-8.46731860157208E-47,6.16297582203915E-33));
#111237=DIRECTION('center_axis',(8.40594773455218E-47,-1.,-9.9579925010296E-17));
#111238=DIRECTION('ref_axis',(-0.923879532511287,-3.81075874975982E-17,
0.382683432365088));
#111239=DIRECTION('center_axis',(-8.40594773455218E-47,1.,9.9579925010296E-17));
#111240=DIRECTION('ref_axis',(-0.923879532511287,-3.81075874975982E-17,
0.382683432365088));
#111241=DIRECTION('',(-8.40594773455218E-47,1.,9.9579925010296E-17));
#111242=DIRECTION('',(8.40594773455218E-47,-1.,-9.9579925010296E-17));
#111243=DIRECTION('center_axis',(-0.707106781186549,-7.04136402448281E-17,
0.707106781186547));
#111244=DIRECTION('ref_axis',(8.40594773455218E-47,-1.,-9.9579925010296E-17));
#111245=DIRECTION('',(0.707106781186546,-7.04136402448283E-17,0.707106781186548));
#111246=DIRECTION('',(8.40594773455218E-47,-1.,-9.9579925010296E-17));
#111247=DIRECTION('center_axis',(-8.40594773455218E-47,1.,9.9579925010296E-17));
#111248=DIRECTION('ref_axis',(-1.,-8.46731860157208E-47,6.16297582203915E-33));
#111249=DIRECTION('',(-1.,-8.46731860157208E-47,6.16297582203915E-33));
#111250=DIRECTION('center_axis',(-8.40594773455218E-47,1.,9.9579925010296E-17));
#111251=DIRECTION('ref_axis',(-0.38268343236509,-9.19998545660213E-17,0.923879532511287));
#111252=DIRECTION('',(8.88178419700125E-16,9.9579925010296E-17,-1.));
#111253=DIRECTION('',(-0.707106781186551,7.04136402448278E-17,-0.707106781186544));
#111254=DIRECTION('center_axis',(8.40594773455218E-47,-1.,-9.9579925010296E-17));
#111255=DIRECTION('ref_axis',(0.0625000000000002,9.93852426637541E-17,-0.998044963916957));
#111256=DIRECTION('center_axis',(8.40594773455218E-47,-1.,-9.9579925010296E-17));
#111257=DIRECTION('ref_axis',(1.,8.46731860157208E-47,-6.16297582203915E-33));
#111258=DIRECTION('center_axis',(8.40594773455218E-47,-1.,-9.9579925010296E-17));
#111259=DIRECTION('ref_axis',(0.12,-9.88603496856012E-17,0.992773891679268));
#111260=DIRECTION('',(6.16297582203915E-33,-9.9579925010296E-17,1.));
#111261=DIRECTION('center_axis',(-8.40594773455218E-47,1.,9.9579925010296E-17));
#111262=DIRECTION('ref_axis',(-1.,-8.46731860157208E-47,6.16297582203915E-33));
#111263=DIRECTION('center_axis',(-8.40594773455218E-47,1.,9.9579925010296E-17));
#111264=DIRECTION('ref_axis',(-0.38268343236509,-9.19998545660213E-17,0.923879532511287));
#111265=DIRECTION('',(-8.40594773455218E-47,1.,9.9579925010296E-17));
#111266=DIRECTION('center_axis',(1.,-8.84447404295016E-32,8.88178419700125E-16));
#111267=DIRECTION('ref_axis',(8.88178419700125E-16,9.9579925010296E-17,
-1.));
#111268=DIRECTION('',(-8.40594773455218E-47,1.,9.9579925010296E-17));
#111269=DIRECTION('center_axis',(0.707106781186544,7.04136402448285E-17,
-0.707106781186551));
#111270=DIRECTION('ref_axis',(-0.707106781186551,7.04136402448278E-17,-0.707106781186544));
#111271=DIRECTION('center_axis',(-0.707106781186544,-7.04136402448285E-17,
0.707106781186551));
#111272=DIRECTION('ref_axis',(-0.707106781186551,7.04136402448278E-17,-0.707106781186544));
#111273=DIRECTION('center_axis',(-1.,-8.46731860157208E-47,6.16297582203915E-33));
#111274=DIRECTION('ref_axis',(-8.40594773455218E-47,1.,9.9579925010296E-17));
#111275=DIRECTION('',(-1.,-8.46731860157208E-47,6.16297582203915E-33));
#111276=DIRECTION('center_axis',(1.,8.46731860157208E-47,-6.16297582203915E-33));
#111277=DIRECTION('ref_axis',(-8.40594773455218E-47,1.,9.9579925010296E-17));
#111278=DIRECTION('',(-1.,-8.46731860157208E-47,6.16297582203915E-33));
#111279=DIRECTION('center_axis',(1.,8.46731860157208E-47,-6.16297582203915E-33));
#111280=DIRECTION('ref_axis',(-8.40594773455218E-47,1.,9.9579925010296E-17));
#111281=DIRECTION('',(0.707106781186548,0.707106781186548,7.04136402448282E-17));
#111282=DIRECTION('',(-0.707106781186548,0.707106781186548,7.04136402448282E-17));
#111283=DIRECTION('center_axis',(-1.,-8.46731860157208E-47,6.16297582203915E-33));
#111284=DIRECTION('ref_axis',(-8.40594773455218E-47,1.,9.9579925010296E-17));
#111285=DIRECTION('center_axis',(0.707106781186548,-0.707106781186548,-7.04136402448282E-17));
#111286=DIRECTION('ref_axis',(0.707106781186548,0.707106781186548,7.04136402448282E-17));
#111287=DIRECTION('',(0.707106781186548,0.707106781186548,7.04136402448282E-17));
#111288=DIRECTION('',(-6.16297582203915E-33,9.9579925010296E-17,-1.));
#111289=DIRECTION('center_axis',(1.,8.46731860157208E-47,-6.16297582203915E-33));
#111290=DIRECTION('ref_axis',(8.40594773455218E-47,-1.,-9.9579925010296E-17));
#111291=DIRECTION('',(0.707106781186548,-0.707106781186548,-7.04136402448282E-17));
#111292=DIRECTION('center_axis',(-1.,-8.46731860157208E-47,6.16297582203915E-33));
#111293=DIRECTION('ref_axis',(8.40594773455218E-47,-1.,-9.9579925010296E-17));
#111294=DIRECTION('center_axis',(0.707106781186544,0.707106781186551,7.04136402448286E-17));
#111295=DIRECTION('ref_axis',(-0.707106781186551,0.707106781186544,7.04136402448278E-17));
#111296=DIRECTION('',(6.16297582203915E-33,-9.9579925010296E-17,1.));
#111297=DIRECTION('center_axis',(-8.40594773455218E-47,1.,9.9579925010296E-17));
#111298=DIRECTION('ref_axis',(-6.16297582203915E-33,9.9579925010296E-17,
-1.));
#111299=DIRECTION('',(-1.,-8.46731860157208E-47,6.16297582203915E-33));
#111300=DIRECTION('',(-6.16297582203915E-33,9.9579925010296E-17,-1.));
#111301=DIRECTION('',(-1.,-8.46731860157208E-47,6.16297582203915E-33));
#111302=DIRECTION('center_axis',(-1.,-8.46731860157208E-47,6.16297582203915E-33));
#111303=DIRECTION('ref_axis',(-8.40594773455218E-47,1.,9.9579925010296E-17));
#111304=DIRECTION('',(-1.,-8.46731860157208E-47,6.16297582203915E-33));
#111305=DIRECTION('center_axis',(-1.,-8.46731860157208E-47,6.16297582203915E-33));
#111306=DIRECTION('ref_axis',(-8.40594773455218E-47,1.,9.9579925010296E-17));
#111307=DIRECTION('center_axis',(8.40594773455218E-47,-1.,-9.9579925010296E-17));
#111308=DIRECTION('ref_axis',(6.16297582203915E-33,-9.9579925010296E-17,
1.));
#111309=DIRECTION('',(-1.,-8.46731860157208E-47,6.16297582203915E-33));
#111310=DIRECTION('',(6.16297582203915E-33,-9.9579925010296E-17,1.));
#111311=DIRECTION('center_axis',(-1.,-8.46731860157208E-47,6.16297582203915E-33));
#111312=DIRECTION('ref_axis',(8.40594773455218E-47,-1.,-9.9579925010296E-17));
#111313=DIRECTION('center_axis',(-1.,-8.46731860157208E-47,6.16297582203915E-33));
#111314=DIRECTION('ref_axis',(8.40594773455218E-47,-1.,-9.9579925010296E-17));
#111315=DIRECTION('center_axis',(1.,8.46731860157208E-47,-6.16297582203915E-33));
#111316=DIRECTION('ref_axis',(6.16297582203915E-33,-9.9579925010296E-17,
1.));
#111317=DIRECTION('',(6.16297582203915E-33,-9.9579925010296E-17,1.));
#111318=DIRECTION('center_axis',(1.,8.46731860157208E-47,-6.16297582203915E-33));
#111319=DIRECTION('ref_axis',(8.40594773455218E-47,-1.,-9.9579925010296E-17));
#111320=DIRECTION('',(-6.16297582203915E-33,9.9579925010296E-17,-1.));
#111321=DIRECTION('center_axis',(-8.40594773455218E-47,1.,9.9579925010296E-17));
#111322=DIRECTION('ref_axis',(-6.16297582203915E-33,9.9579925010296E-17,
-1.));
#111323=DIRECTION('',(-1.,-8.46731860157208E-47,6.16297582203915E-33));
#111324=DIRECTION('center_axis',(8.40594773455218E-47,-1.,-9.9579925010296E-17));
#111325=DIRECTION('ref_axis',(6.16297582203915E-33,-9.9579925010296E-17,
1.));
#111326=DIRECTION('',(-1.,-8.46731860157208E-47,6.16297582203915E-33));
#111327=DIRECTION('center_axis',(-1.,-8.46731860157208E-47,6.16297582203915E-33));
#111328=DIRECTION('ref_axis',(8.40594773455218E-47,-1.,-9.9579925010296E-17));
#111329=DIRECTION('center_axis',(8.40594773455218E-47,-1.,-9.9579925010296E-17));
#111330=DIRECTION('ref_axis',(1.,8.46731860157208E-47,-6.16297582203915E-33));
#111331=DIRECTION('center_axis',(-8.40594773455218E-47,1.,9.9579925010296E-17));
#111332=DIRECTION('ref_axis',(1.,8.46731860157208E-47,-6.16297582203915E-33));
#111333=DIRECTION('center_axis',(-8.40594773455218E-47,1.,9.9579925010296E-17));
#111334=DIRECTION('ref_axis',(1.,8.46731860157208E-47,-6.16297582203915E-33));
#111335=DIRECTION('center_axis',(8.40594773455218E-47,-1.,-9.9579925010296E-17));
#111336=DIRECTION('ref_axis',(1.,8.46731860157208E-47,-6.16297582203915E-33));
#111337=DIRECTION('center_axis',(-8.40594773455218E-47,1.,9.9579925010296E-17));
#111338=DIRECTION('ref_axis',(-1.,-8.46731860157208E-47,6.16297582203915E-33));
#111339=DIRECTION('',(6.16297582203915E-33,-9.9579925010296E-17,1.));
#111340=DIRECTION('center_axis',(-8.40594773455218E-47,1.,9.9579925010296E-17));
#111341=DIRECTION('ref_axis',(-1.,-1.56620894510576E-31,1.5728159515523E-15));
#111342=DIRECTION('center_axis',(-8.40594773455218E-47,1.,9.9579925010296E-17));
#111343=DIRECTION('ref_axis',(-0.449999999999999,8.89277165364225E-17,-0.893028554974588));
#111344=DIRECTION('center_axis',(8.40594773455218E-47,-1.,-9.9579925010296E-17));
#111345=DIRECTION('ref_axis',(1.,8.46731860157207E-47,-6.16297582203915E-33));
#111346=DIRECTION('center_axis',(8.40594773455218E-47,-1.,-9.9579925010296E-17));
#111347=DIRECTION('ref_axis',(1.,8.46731860157208E-47,-6.16297582203915E-33));
#111348=DIRECTION('center_axis',(8.40594773455218E-47,-1.,-9.9579925010296E-17));
#111349=DIRECTION('ref_axis',(-1.,-1.56620894510576E-31,1.5728159515523E-15));
#111350=DIRECTION('',(-6.16297582203915E-33,9.9579925010296E-17,-1.));
#111351=DIRECTION('center_axis',(8.40594773455218E-47,-1.,-9.9579925010296E-17));
#111352=DIRECTION('ref_axis',(-0.449999999999999,8.89277165364225E-17,-0.893028554974588));
#111353=DIRECTION('center_axis',(-8.40594773455218E-47,1.,9.9579925010296E-17));
#111354=DIRECTION('ref_axis',(1.,8.46731860157207E-47,-6.16297582203915E-33));
#111355=DIRECTION('center_axis',(8.40594773455218E-47,-1.,-9.9579925010296E-17));
#111356=DIRECTION('ref_axis',(1.,8.46731860157208E-47,-6.16297582203915E-33));
#111357=DIRECTION('center_axis',(-8.40594773455218E-47,1.,9.9579925010296E-17));
#111358=DIRECTION('ref_axis',(1.,8.46731860157208E-47,-6.16297582203915E-33));
#111359=DIRECTION('center_axis',(-8.40594773455218E-47,1.,9.9579925010296E-17));
#111360=DIRECTION('ref_axis',(1.,8.46731860157208E-47,-6.16297582203915E-33));
#111361=DIRECTION('center_axis',(8.40594773455218E-47,-1.,-9.9579925010296E-17));
#111362=DIRECTION('ref_axis',(1.,8.46731860157208E-47,-6.16297582203915E-33));
#111363=DIRECTION('center_axis',(8.40594773455218E-47,-1.,-9.9579925010296E-17));
#111364=DIRECTION('ref_axis',(1.,8.46731860157208E-47,-6.16297582203915E-33));
#111365=DIRECTION('',(-6.16297582203915E-33,9.9579925010296E-17,-1.));
#111366=DIRECTION('center_axis',(8.40594773455218E-47,-1.,-9.9579925010296E-17));
#111367=DIRECTION('ref_axis',(-0.449999999999999,8.89277165364225E-17,-0.893028554974588));
#111368=DIRECTION('center_axis',(8.40594773455218E-47,-1.,-9.9579925010296E-17));
#111369=DIRECTION('ref_axis',(-1.,-1.56620894510576E-31,1.5728159515523E-15));
#111370=DIRECTION('center_axis',(-8.40594773455218E-47,1.,9.9579925010296E-17));
#111371=DIRECTION('ref_axis',(1.,8.46731860157207E-47,-6.16297582203915E-33));
#111372=DIRECTION('center_axis',(-8.40594773455218E-47,1.,9.9579925010296E-17));
#111373=DIRECTION('ref_axis',(1.,8.46731860157208E-47,-6.16297582203915E-33));
#111374=DIRECTION('center_axis',(-8.40594773455218E-47,1.,9.9579925010296E-17));
#111375=DIRECTION('ref_axis',(-1.,-1.56620894510576E-31,1.5728159515523E-15));
#111376=DIRECTION('center_axis',(-8.40594773455218E-47,1.,9.9579925010296E-17));
#111377=DIRECTION('ref_axis',(-0.449999999999999,8.89277165364225E-17,-0.893028554974588));
#111378=DIRECTION('',(6.16297582203915E-33,-9.9579925010296E-17,1.));
#111379=DIRECTION('center_axis',(8.40594773455218E-47,-1.,-9.9579925010296E-17));
#111380=DIRECTION('ref_axis',(1.,8.46731860157207E-47,-6.16297582203915E-33));
#111381=DIRECTION('center_axis',(8.40594773455218E-47,-1.,-9.9579925010296E-17));
#111382=DIRECTION('ref_axis',(0.0625000000000002,9.93852426637541E-17,-0.998044963916957));
#111383=DIRECTION('',(8.40594773455218E-47,-1.,-9.9579925010296E-17));
#111384=DIRECTION('center_axis',(8.40594773455218E-47,-1.,-9.9579925010296E-17));
#111385=DIRECTION('ref_axis',(-0.85146931829632,5.22201532254593E-17,-0.524404424085075));
#111386=DIRECTION('',(-8.40594773455218E-47,1.,9.9579925010296E-17));
#111387=DIRECTION('',(8.40594773455218E-47,-1.,-9.9579925010296E-17));
#111388=DIRECTION('center_axis',(-1.,-8.46731860157208E-47,6.16297582203915E-33));
#111389=DIRECTION('ref_axis',(-6.16297582203915E-33,9.9579925010296E-17,
-1.));
#111390=DIRECTION('',(8.40594773455218E-47,-1.,-9.9579925010296E-17));
#111391=DIRECTION('center_axis',(8.40594773455218E-47,-1.,-9.9579925010296E-17));
#111392=DIRECTION('ref_axis',(-0.811844140885989,-5.81421498601493E-17,
0.583874208121142));
#111393=DIRECTION('center_axis',(8.40594773455218E-47,-1.,-9.9579925010296E-17));
#111394=DIRECTION('ref_axis',(1.,8.46731860157208E-47,-6.16297582203915E-33));
#111395=DIRECTION('center_axis',(8.40594773455218E-47,-1.,-9.9579925010296E-17));
#111396=DIRECTION('ref_axis',(-1.,-8.46731860157208E-47,6.16297582203915E-33));
#111397=DIRECTION('center_axis',(-8.40594773455218E-47,1.,9.9579925010296E-17));
#111398=DIRECTION('ref_axis',(-1.,-8.46731860157207E-47,6.16297582203915E-33));
#111399=DIRECTION('center_axis',(-8.40594773455218E-47,1.,9.9579925010296E-17));
#111400=DIRECTION('ref_axis',(-1.,-8.46731860157208E-47,6.16297582203915E-33));
#111401=DIRECTION('center_axis',(-8.40594773455218E-47,1.,9.9579925010296E-17));
#111402=DIRECTION('ref_axis',(-1.,-8.46731860157208E-47,6.16297582203915E-33));
#111403=DIRECTION('',(-0.898876371703422,4.36361536127186E-17,-0.438202314454514));
#111404=DIRECTION('center_axis',(-8.40594773455218E-47,1.,9.9579925010296E-17));
#111405=DIRECTION('ref_axis',(-1.,-8.46731860157208E-47,6.16297582203915E-33));
#111406=DIRECTION('center_axis',(-8.40594773455218E-47,1.,9.9579925010296E-17));
#111407=DIRECTION('ref_axis',(-1.,-8.46731860157208E-47,6.16297582203915E-33));
#111408=DIRECTION('center_axis',(8.40594773455218E-47,-1.,-9.9579925010296E-17));
#111409=DIRECTION('ref_axis',(-1.,-8.46731860157207E-47,6.16297582203915E-33));
#111410=DIRECTION('center_axis',(8.40594773455218E-47,-1.,-9.9579925010296E-17));
#111411=DIRECTION('ref_axis',(-1.,-8.46731860157208E-47,6.16297582203915E-33));
#111412=DIRECTION('center_axis',(8.40594773455218E-47,-1.,-9.9579925010296E-17));
#111413=DIRECTION('ref_axis',(-1.,-8.46731860157208E-47,6.16297582203915E-33));
#111414=DIRECTION('',(-0.898876371703422,4.36361536127186E-17,-0.438202314454514));
#111415=DIRECTION('center_axis',(-1.,-8.46731860157208E-47,6.16297582203915E-33));
#111416=DIRECTION('ref_axis',(-6.16297582203915E-33,9.9579925010296E-17,
-1.));
#111417=DIRECTION('',(8.40594773455218E-47,-1.,-9.9579925010296E-17));
#111418=DIRECTION('',(8.40594773455218E-47,-1.,-9.9579925010296E-17));
#111419=DIRECTION('center_axis',(-1.,-8.46731860157208E-47,6.16297582203915E-33));
#111420=DIRECTION('ref_axis',(-6.16297582203915E-33,9.9579925010296E-17,
-1.));
#111421=DIRECTION('',(-8.40594773455218E-47,1.,9.9579925010296E-17));
#111422=DIRECTION('',(8.40594773455218E-47,-1.,-9.9579925010296E-17));
#111423=DIRECTION('center_axis',(-8.40594773455218E-47,1.,9.9579925010296E-17));
#111424=DIRECTION('ref_axis',(0.12,-9.88603496856012E-17,0.992773891679268));
#111425=DIRECTION('center_axis',(-8.40594773455218E-47,1.,9.9579925010296E-17));
#111426=DIRECTION('ref_axis',(0.12,-9.88603496856012E-17,0.992773891679268));
#111427=DIRECTION('',(8.40594773455218E-47,-1.,-9.9579925010296E-17));
#111428=DIRECTION('center_axis',(8.40594773455218E-47,-1.,-9.9579925010296E-17));
#111429=DIRECTION('ref_axis',(-0.85146931829632,5.22201532254593E-17,-0.524404424085075));
#111430=DIRECTION('center_axis',(8.40594773455218E-47,-1.,-9.9579925010296E-17));
#111431=DIRECTION('ref_axis',(-1.,-8.46731860157207E-47,6.16297582203915E-33));
#111432=DIRECTION('',(-8.40594773455218E-47,1.,9.9579925010296E-17));
#111433=DIRECTION('center_axis',(8.40594773455218E-47,-1.,-9.9579925010296E-17));
#111434=DIRECTION('ref_axis',(-0.811844140885989,-5.81421498601493E-17,
0.583874208121142));
#111435=DIRECTION('center_axis',(6.16297582203915E-33,-9.9579925010296E-17,
1.));
#111436=DIRECTION('ref_axis',(-1.,-8.46731860157208E-47,6.16297582203915E-33));
#111437=DIRECTION('center_axis',(0.438202314454514,8.95100416877536E-17,
-0.898876371703421));
#111438=DIRECTION('ref_axis',(0.898876371703422,-4.36361536127186E-17,0.438202314454514));
#111439=DIRECTION('',(8.40594773455218E-47,-1.,-9.9579925010296E-17));
#111440=DIRECTION('center_axis',(8.40594773455218E-47,-1.,-9.9579925010296E-17));
#111441=DIRECTION('ref_axis',(-1.,-8.46731860157207E-47,6.16297582203915E-33));
#111442=DIRECTION('',(-8.40594773455218E-47,1.,9.9579925010296E-17));
#111443=DIRECTION('center_axis',(8.40594773455218E-47,-1.,-9.9579925010296E-17));
#111444=DIRECTION('ref_axis',(-1.,-8.46731860157207E-47,6.16297582203915E-33));
#111445=DIRECTION('',(-8.40594773455218E-47,1.,9.9579925010296E-17));
#111446=DIRECTION('center_axis',(8.40594773455218E-47,-1.,-9.9579925010296E-17));
#111447=DIRECTION('ref_axis',(-1.,-8.46731860157208E-47,6.16297582203915E-33));
#111448=DIRECTION('',(-8.40594773455218E-47,1.,9.9579925010296E-17));
#111449=DIRECTION('',(-8.40594773455218E-47,1.,9.9579925010296E-17));
#145398=CARTESIAN_POINT('',(0.,0.,0.));
#145399=CARTESIAN_POINT('Origin',(3.99999981302311,0.199999999999988,2.50184806546842));
#145400=CARTESIAN_POINT('',(3.99999981302311,11.9,2.50184806546842));
#145401=CARTESIAN_POINT('',(-0.600000000002621,11.9,7.10184787849414));
#145402=CARTESIAN_POINT('',(-0.849538123856316,11.9,7.35138600234784));
#145403=CARTESIAN_POINT('',(3.99999981302311,14.4,2.50184806546842));
#145404=CARTESIAN_POINT('',(3.99999957308175,7.29999999999999,2.50184830540978));
#145405=CARTESIAN_POINT('',(-0.600000000002621,14.4,7.10184787849414));
#145406=CARTESIAN_POINT('',(-1.18078817722572,14.4,7.68263605571724));
#145407=CARTESIAN_POINT('',(-0.600000000002621,0.199999999999988,7.10184787849414));
#145408=CARTESIAN_POINT('Origin',(3.99999981302311,0.199999999999988,2.50184806546842));
#145409=CARTESIAN_POINT('',(-0.600000000002621,2.1,7.10184787849414));
#145410=CARTESIAN_POINT('',(3.99999981302311,2.1,2.50184806546842));
#145411=CARTESIAN_POINT('',(-0.849538123856316,2.1,7.35138600234784));
#145412=CARTESIAN_POINT('',(-0.600000000002621,0.199999999999988,7.10184787849414));
#145413=CARTESIAN_POINT('',(-0.600000000002621,0.199999999999988,7.10184787849414));
#145414=CARTESIAN_POINT('',(3.99999981302311,0.199999999999988,2.50184806546842));
#145415=CARTESIAN_POINT('',(-1.18078817722572,0.199999999999988,7.68263605571724));
#145416=CARTESIAN_POINT('',(3.99999957308175,7.29999999999999,2.50184830540978));
#145417=CARTESIAN_POINT('Origin',(-2.20000021345912,14.4,17.0249999999815));
#145418=CARTESIAN_POINT('',(-0.599999999994357,14.4,15.0499999999722));
#145419=CARTESIAN_POINT('',(-0.600000000010333,14.4,12.0634239392391));
#145420=CARTESIAN_POINT('',(3.99999957308175,14.4,0.00184806546839056));
#145421=CARTESIAN_POINT('',(3.99999957308175,14.4,-4.44089209850063E-15));
#145422=CARTESIAN_POINT('',(-3.99999999999999,14.4,-4.44089209850063E-15));
#145423=CARTESIAN_POINT('Origin',(1.33226762955019E-14,14.4,-4.44089209850063E-15));
#145424=CARTESIAN_POINT('',(-3.99999999999999,14.4,3.08613054156667));
#145425=CARTESIAN_POINT('',(-3.99999999999999,14.4,-4.44089209850063E-15));
#145426=CARTESIAN_POINT('',(-6.0957241205081,14.4,7.15616513795545));
#145427=CARTESIAN_POINT('Origin',(-8.99999999999999,14.4,3.08613054156667));
#145428=CARTESIAN_POINT('',(-5.25380888164337,14.4,16.9135949821128));
#145429=CARTESIAN_POINT('Origin',(-5.84999999999999,14.4,12.049999999963));
#145430=CARTESIAN_POINT('',(-0.899999999999987,14.4,24.0343597112987));
#145431=CARTESIAN_POINT('Origin',(-8.89999999999999,14.4,24.0343597112987));
#145432=CARTESIAN_POINT('',(-0.899999999999987,14.4,32.4000004268813));
#145433=CARTESIAN_POINT('',(-0.899999999999987,14.4,16.049999999963));
#145434=CARTESIAN_POINT('',(-4.26918251861252E-7,14.4,33.299999999963));
#145435=CARTESIAN_POINT('',(-4.61875037354885,14.4,28.6812500533325));
#145436=CARTESIAN_POINT('',(-4.26918254081698E-7,14.4,36.3857864375899));
#145437=CARTESIAN_POINT('',(-4.2691824742036E-7,14.4,27.6624999999723));
#145438=CARTESIAN_POINT('',(0.292892791895201,14.4,37.0928932187765));
#145439=CARTESIAN_POINT('Origin',(0.999999573081747,14.4,36.3857864375899));
#145440=CARTESIAN_POINT('',(1.20710635426829,14.4,38.0071067811496));
#145441=CARTESIAN_POINT('',(-5.11875037354885,14.4,31.6812500533324));
#145442=CARTESIAN_POINT('',(1.91421313545483,14.4,38.299999999963));
#145443=CARTESIAN_POINT('Origin',(1.91421313545483,14.4,37.299999999963));
#145444=CARTESIAN_POINT('',(3.99999957308175,14.4,38.299999999963));
#145445=CARTESIAN_POINT('',(0.899999679811312,14.4,38.299999999963));
#145446=CARTESIAN_POINT('',(4.,14.4,19.6499999999665));
#145447=CARTESIAN_POINT('',(3.99999957308175,14.4,-4.44089209850063E-15));
#145448=CARTESIAN_POINT('',(0.493749946643665,14.4,16.1437499466102));
#145449=CARTESIAN_POINT('Origin',(-5.84999999999999,2.1,12.049999999963));
#145450=CARTESIAN_POINT('',(-0.599999999994357,2.09999999999999,15.0499999999722));
#145451=CARTESIAN_POINT('',(-0.600000000006467,2.1,9.57592393923266));
#145452=CARTESIAN_POINT('',(1.75042009953066,2.1,3.59666921959181));
#145453=CARTESIAN_POINT('',(-2.98516557716169,2.1,5.90137500303677));
#145454=CARTESIAN_POINT('',(0.461099356094962,2.09999999999999,3.97333454214578));
#145455=CARTESIAN_POINT('Origin',(1.33226762955019E-14,2.09999999999999,
-2.49800183849383E-15));
#145456=CARTESIAN_POINT('',(-3.40729205497977,2.09999999999999,2.09531879485477));
#145457=CARTESIAN_POINT('Origin',(-5.84999999999999,2.1,12.049999999963));
#145458=CARTESIAN_POINT('',(-3.99999999999999,2.09999999999999,-1.99840144432528E-13));
#145459=CARTESIAN_POINT('Origin',(1.33226762955019E-14,2.09999999999999,
-2.49800183849383E-15));
#145460=CARTESIAN_POINT('',(-3.99999999999999,2.1,3.08613054156667));
#145461=CARTESIAN_POINT('',(-3.99999999999999,2.09999999999999,9.87500000569498));
#145462=CARTESIAN_POINT('',(-6.74999999999999,2.1,7.5512733164396));
#145463=CARTESIAN_POINT('Origin',(-8.99999999999999,2.1,3.08613054156667));
#145464=CARTESIAN_POINT('',(-7.66385919120079,2.1,8.26187185607765));
#145465=CARTESIAN_POINT('Origin',(-5.39999999999999,2.1,10.2303589813634));
#145466=CARTESIAN_POINT('',(-7.1474157554001,2.1,16.0445853799042));
#145467=CARTESIAN_POINT('Origin',(-5.84999999999999,2.1,12.049999999963));
#145468=CARTESIAN_POINT('',(-6.35454545454544,2.1,16.4501220332571));
#145469=CARTESIAN_POINT('Origin',(-5.39999999999999,2.1,13.6060329039916));
#145470=CARTESIAN_POINT('',(-0.899999999999982,2.09999999999999,24.0343597112987));
#145471=CARTESIAN_POINT('Origin',(-8.89999999999999,2.09999999999999,24.0343597112987));
#145472=CARTESIAN_POINT('',(-0.899999999999987,2.09999999999999,25.399999999963));
#145473=CARTESIAN_POINT('',(-0.899999999999987,2.09999999999999,25.049999999963));
#145474=CARTESIAN_POINT('',(1.10000000000001,2.09999999999999,23.399999999963));
#145475=CARTESIAN_POINT('',(1.70000000000002,2.09999999999999,22.799999999963));
#145476=CARTESIAN_POINT('',(4.,2.09999999999999,23.399999999963));
#145477=CARTESIAN_POINT('',(3.,2.09999999999999,23.399999999963));
#145478=CARTESIAN_POINT('',(4.,2.09999999999999,19.6499999999665));
#145479=CARTESIAN_POINT('',(3.99999957308175,2.09999999999999,10.4499999999815));
#145480=CARTESIAN_POINT('',(3.38750000000382,2.09999999999999,19.0374999999704));
#145481=CARTESIAN_POINT('Origin',(1.75042009953066,0.199999999999991,3.59666921959181));
#145482=CARTESIAN_POINT('',(3.99999957308175,8.24999999999999,2.50184818224262));
#145483=CARTESIAN_POINT('',(1.75042009953066,11.9,3.59666921959181));
#145484=CARTESIAN_POINT('',(3.92607865052219,11.9,2.53782387550884));
#145485=CARTESIAN_POINT('',(1.75042009953066,11.9,3.59666921959181));
#145486=CARTESIAN_POINT('Origin',(-5.84999999999999,11.9,12.049999999963));
#145487=CARTESIAN_POINT('',(-0.599999999994357,11.9,15.0499999999722));
#145488=CARTESIAN_POINT('',(-0.600000000006467,11.9,9.57592393923266));
#145489=CARTESIAN_POINT('',(4.,11.9,19.6499999999665));
#145490=CARTESIAN_POINT('',(2.2000000000047,11.9,17.8499999999712));
#145491=CARTESIAN_POINT('',(4.,11.9,23.399999999963));
#145492=CARTESIAN_POINT('',(3.99999957308175,11.9,8.07499999998326));
#145493=CARTESIAN_POINT('',(1.10000000000001,11.9,23.399999999963));
#145494=CARTESIAN_POINT('',(1.99999957308175,11.9,23.399999999963));
#145495=CARTESIAN_POINT('',(-0.899999999999987,11.9,25.399999999963));
#145496=CARTESIAN_POINT('',(1.70000000000002,11.9,22.799999999963));
#145497=CARTESIAN_POINT('',(-0.899999999999982,11.9,24.0343597112987));
#145498=CARTESIAN_POINT('',(-0.899999999999987,11.9,25.049999999963));
#145499=CARTESIAN_POINT('',(-6.35454545454544,11.9,16.4501220332571));
#145500=CARTESIAN_POINT('Origin',(-8.89999999999999,11.9,24.0343597112987));
#145501=CARTESIAN_POINT('',(-7.1474157554001,11.9,16.0445853799042));
#145502=CARTESIAN_POINT('Origin',(-5.39999999999999,11.9,13.6060329039916));
#145503=CARTESIAN_POINT('',(-7.66385919120079,11.9,8.26187185607765));
#145504=CARTESIAN_POINT('Origin',(-5.84999999999999,11.9,12.049999999963));
#145505=CARTESIAN_POINT('',(-6.74999999999999,11.9,7.55127331643961));
#145506=CARTESIAN_POINT('Origin',(-5.39999999999999,11.9,10.2303589813634));
#145507=CARTESIAN_POINT('',(-3.99999999999999,11.9,3.08613054156667));
#145508=CARTESIAN_POINT('Origin',(-8.99999999999999,11.9,3.08613054156667));
#145509=CARTESIAN_POINT('',(-3.99999999999999,11.9,-2.00427047043497E-13));
#145510=CARTESIAN_POINT('',(-3.99999999999999,11.9,9.87500000569498));
#145511=CARTESIAN_POINT('',(-3.40729205497977,11.9,2.09531879485477));
#145512=CARTESIAN_POINT('Origin',(1.33226762955019E-14,11.9,-2.49800183849383E-15));
#145513=CARTESIAN_POINT('',(0.461099356094962,11.9,3.97333454214578));
#145514=CARTESIAN_POINT('Origin',(-5.84999999999999,11.9,12.049999999963));
#145515=CARTESIAN_POINT('Origin',(1.33226762955019E-14,11.9,-2.49800183849383E-15));
#145516=CARTESIAN_POINT('Origin',(0.100000000000013,13.15,24.399999999963));
#145517=CARTESIAN_POINT('',(1.10000000000001,13.15,23.399999999963));
#145518=CARTESIAN_POINT('',(-0.899999999999987,13.15,25.399999999963));
#145519=CARTESIAN_POINT('Origin',(-0.899999999999987,14.4,38.049999999963));
#145520=CARTESIAN_POINT('',(-0.899999999999987,0.199999999999987,24.0343597112987));
#145521=CARTESIAN_POINT('',(-0.899999999999987,14.4,24.0343597112987));
#145522=CARTESIAN_POINT('',(-0.899999999999987,0.199999999999982,32.4000004268813));
#145523=CARTESIAN_POINT('',(-0.899999999999987,0.199999999999982,27.5374999999723));
#145524=CARTESIAN_POINT('',(-0.899999999999987,6.72554492441848,32.4000004268813));
#145525=CARTESIAN_POINT('',(-0.899999999999987,7.29999999999999,32.4000004268813));
#145526=CARTESIAN_POINT('',(-0.900000426918255,5.59999999999999,30.799999999963));
#145527=CARTESIAN_POINT('Origin',(-0.899999999999987,7.29999999999998,30.799999999963));
#145528=CARTESIAN_POINT('',(-0.900000426918255,5.59999999999999,27.799999999963));
#145529=CARTESIAN_POINT('',(-0.899999999999987,5.59999999999999,32.924999999963));
#145530=CARTESIAN_POINT('',(-0.900000426918255,8.99999999999999,27.799999999963));
#145531=CARTESIAN_POINT('Origin',(-0.899999999999987,7.29999999999999,27.799999999963));
#145532=CARTESIAN_POINT('',(-0.900000426918255,8.99999999999998,30.799999999963));
#145533=CARTESIAN_POINT('',(-0.899999999999987,8.99999999999998,34.424999999963));
#145534=CARTESIAN_POINT('',(-0.899999999999987,7.87445507558149,32.4000004268813));
#145535=CARTESIAN_POINT('Origin',(-0.899999999999987,7.29999999999998,30.799999999963));
#145536=CARTESIAN_POINT('',(-0.899999999999987,7.29999999999999,32.4000004268813));
#145537=CARTESIAN_POINT('',(-0.899999999999987,14.4,24.0343597112987));
#145538=CARTESIAN_POINT('Origin',(3.99999957308175,14.4,-2.5));
#145539=CARTESIAN_POINT('',(3.99999957308175,13.15,23.399999999963));
#145540=CARTESIAN_POINT('',(3.99999957308175,6.09999999999999,19.6499995730483));
#145541=CARTESIAN_POINT('',(3.99999957308175,0.199999999999987,38.299999999963));
#145542=CARTESIAN_POINT('',(3.99999957308175,14.4,38.299999999963));
#145543=CARTESIAN_POINT('',(4.,0.199999999999987,19.6499999999665));
#145544=CARTESIAN_POINT('',(3.99999957308175,0.199999999999987,7.26249999999075));
#145545=CARTESIAN_POINT('',(3.99999957308175,6.09999999999999,19.6499995730483));
#145546=CARTESIAN_POINT('',(3.99999957308175,10.7,30.799999999963));
#145547=CARTESIAN_POINT('',(3.99999957308175,3.89999999999998,30.799999999963));
#145548=CARTESIAN_POINT('Origin',(3.99999957308175,7.29999999999998,30.799999999963));
#145549=CARTESIAN_POINT('',(3.99999957308175,10.7,27.799999999963));
#145550=CARTESIAN_POINT('',(3.99999957308175,10.7,14.1499999999815));
#145551=CARTESIAN_POINT('',(3.99999957308175,3.89999999999999,27.799999999963));
#145552=CARTESIAN_POINT('Origin',(3.99999957308175,7.29999999999999,27.799999999963));
#145553=CARTESIAN_POINT('',(3.99999957308175,3.89999999999999,12.6499999999815));
#145554=CARTESIAN_POINT('Origin',(1.40000000000941,-2.2,17.0499999999759));
#145555=CARTESIAN_POINT('',(-0.599999999994357,-2.2,15.0499999999722));
#145556=CARTESIAN_POINT('Origin',(1.99999957308175,11.9,23.399999999963));
#145557=CARTESIAN_POINT('Origin',(-8.89999999999999,14.4,24.0343597112987));
#145558=CARTESIAN_POINT('',(-6.35454545129335,14.8710452666677,16.4501220343486));
#145559=CARTESIAN_POINT('Ctrl Pts',(-5.25380888164336,14.4,16.9135949821128));
#145560=CARTESIAN_POINT('Ctrl Pts',(-5.33338146986815,14.4501241917611,
16.8728497987675));
#145561=CARTESIAN_POINT('Ctrl Pts',(-5.41464812969736,14.4979663578989,
16.8329226337617));
#145562=CARTESIAN_POINT('Ctrl Pts',(-5.76835566322084,14.6899428683665,
16.6667013086606));
#145563=CARTESIAN_POINT('Ctrl Pts',(-6.05674662065273,14.8056725793831,
16.5500705618533));
#145564=CARTESIAN_POINT('Ctrl Pts',(-6.35454545128526,14.8710452666659,
16.4501220343513));
#145565=CARTESIAN_POINT('',(-6.35454545454544,14.4,16.4501220332571));
#145566=CARTESIAN_POINT('Origin',(1.33226762955019E-14,11.9,-2.49800183849383E-15));
#145567=CARTESIAN_POINT('',(0.461099356094962,11.9,3.97333454214578));
#145568=CARTESIAN_POINT('Origin',(-3.99999999999999,14.4,8.04999999996301));
#145569=CARTESIAN_POINT('',(-3.99999999999999,14.4,3.08613054156667));
#145570=CARTESIAN_POINT('',(-3.99999999999999,14.4,-4.44089209850063E-15));
#145571=CARTESIAN_POINT('Origin',(-5.84999999999999,11.6,12.049999999963));
#145572=CARTESIAN_POINT('',(-3.40729205497977,11.9,2.09531879485477));
#145573=CARTESIAN_POINT('Origin',(1.40000000000941,-2.2,17.0499999999759));
#145574=CARTESIAN_POINT('',(-0.599999999994357,0.199999999999987,15.0499999999722));
#145575=CARTESIAN_POINT('',(0.493749946643668,0.199999999999987,16.1437499466102));
#145576=CARTESIAN_POINT('',(-0.599999999994357,-2.2,15.0499999999722));
#145577=CARTESIAN_POINT('Origin',(-0.600000000009414,-2.19999999999999,
7.0499999999797));
#145578=CARTESIAN_POINT('',(-0.600000000010333,0.199999999999987,12.0634239392391));
#145579=CARTESIAN_POINT('Origin',(-0.600000000009414,-2.19999999999999,
7.0499999999797));
#145580=CARTESIAN_POINT('Origin',(3.99999957308175,14.4,-2.5));
#145581=CARTESIAN_POINT('',(3.99999957308175,0.199999999999991,0.00184806546839056));
#145582=CARTESIAN_POINT('',(3.99999957308175,0.199999999999987,7.26249999999075));
#145583=CARTESIAN_POINT('',(4.00000000000001,0.199999999999991,-4.44089209850063E-15));
#145584=CARTESIAN_POINT('',(3.99999957308175,0.199999999999987,7.26249999999075));
#145585=CARTESIAN_POINT('',(3.99999957308175,0.199999999999991,-2.5));
#145586=CARTESIAN_POINT('',(3.99999957308175,0.199999999999987,7.26249999999075));
#145587=CARTESIAN_POINT('',(3.99999957308175,14.4,-2.5));
#145588=CARTESIAN_POINT('',(3.99999957308175,14.4,-2.5));
#145589=CARTESIAN_POINT('',(4.00000000000001,14.4,-4.44089209850063E-15));
#145590=CARTESIAN_POINT('',(3.99999957308175,14.4,-4.44089209850063E-15));
#145591=CARTESIAN_POINT('Origin',(1.33226762955019E-14,14.4,-4.44089209850063E-15));
#145592=CARTESIAN_POINT('Origin',(0.999999573081747,3.74999999999998,36.3857864375899));
#145593=CARTESIAN_POINT('',(-4.26918254081698E-7,0.199999999999987,36.3857864375899));
#145594=CARTESIAN_POINT('',(0.292892791895201,0.199999999999987,37.0928932187765));
#145595=CARTESIAN_POINT('Origin',(0.999999573081747,0.199999999999987,36.3857864375899));
#145596=CARTESIAN_POINT('',(0.292892791895198,3.74999999999998,37.0928932187765));
#145597=CARTESIAN_POINT('',(-4.26918254081698E-7,3.74999999999998,36.3857864375899));
#145598=CARTESIAN_POINT('Origin',(0.749999573081743,7.29999999999999,37.549999999963));
#145599=CARTESIAN_POINT('',(1.20710635426829,0.199999999999987,38.0071067811496));
#145600=CARTESIAN_POINT('',(-5.11875037354885,0.199999999999982,31.6812500533324));
#145601=CARTESIAN_POINT('',(1.20710635426828,10.85,38.0071067811496));
#145602=CARTESIAN_POINT('Origin',(-2.20000021345912,0.199999999999987,17.0249999999815));
#145603=CARTESIAN_POINT('',(1.91421313545483,0.199999999999987,38.299999999963));
#145604=CARTESIAN_POINT('',(0.899999679811312,0.199999999999987,38.299999999963));
#145605=CARTESIAN_POINT('Origin',(1.91421313545483,0.199999999999987,37.299999999963));
#145606=CARTESIAN_POINT('',(-4.26918251861252E-7,0.199999999999987,33.299999999963));
#145607=CARTESIAN_POINT('',(-4.2691824742036E-7,0.199999999999982,27.6624999999723));
#145608=CARTESIAN_POINT('',(-4.61875037354885,0.199999999999982,28.6812500533325));
#145609=CARTESIAN_POINT('',(-5.25380888164337,0.199999999999987,16.9135949821128));
#145610=CARTESIAN_POINT('Origin',(-8.89999999999999,0.199999999999987,24.0343597112987));
#145611=CARTESIAN_POINT('',(-6.0957241205081,0.199999999999987,7.15616513795545));
#145612=CARTESIAN_POINT('Origin',(-5.84999999999999,0.199999999999987,12.049999999963));
#145613=CARTESIAN_POINT('',(-3.99999999999999,0.199999999999991,3.08613054156667));
#145614=CARTESIAN_POINT('Origin',(-8.99999999999999,0.199999999999991,3.08613054156667));
#145615=CARTESIAN_POINT('',(-3.99999999999999,0.199999999999991,-4.44089209850063E-15));
#145616=CARTESIAN_POINT('',(-3.99999999999999,0.199999999999987,12.5374999999723));
#145617=CARTESIAN_POINT('Origin',(1.33226762955019E-14,0.199999999999991,
-4.44089209850063E-15));
#145618=CARTESIAN_POINT('Origin',(1.91421313545483,10.85,37.299999999963));
#145619=CARTESIAN_POINT('',(1.91421313545483,10.85,38.299999999963));
#145620=CARTESIAN_POINT('Origin',(-4.26918256302145E-7,0.199999999999987,
38.299999999963));
#145621=CARTESIAN_POINT('',(-4.26918251861252E-7,0.199999999999987,33.299999999963));
#145622=CARTESIAN_POINT('Origin',(-4.26918251861252E-7,0.199999999999987,
33.299999999963));
#145623=CARTESIAN_POINT('Origin',(-2.50000042691827,7.29999999999998,30.799999999963));
#145624=CARTESIAN_POINT('Origin',(3.99999957308175,7.29999999999998,30.799999999963));
#145625=CARTESIAN_POINT('',(1.99999957308175,8.99999999999998,30.799999999963));
#145626=CARTESIAN_POINT('',(3.99999957308175,8.99999999999998,30.799999999963));
#145627=CARTESIAN_POINT('',(1.99999957308175,5.59999999999999,30.799999999963));
#145628=CARTESIAN_POINT('Origin',(1.99999957308175,7.29999999999998,30.799999999963));
#145629=CARTESIAN_POINT('',(3.99999957308175,5.59999999999999,30.799999999963));
#145630=CARTESIAN_POINT('Origin',(3.89999957308174,7.29999999999998,30.799999999963));
#145631=CARTESIAN_POINT('',(3.79999957308174,10.5,30.799999999963));
#145632=CARTESIAN_POINT('',(3.79999957308174,10.5,30.799999999963));
#145633=CARTESIAN_POINT('',(3.79999957308174,4.09999999999998,30.799999999963));
#145634=CARTESIAN_POINT('',(3.99999957308175,3.89999999999998,30.799999999963));
#145635=CARTESIAN_POINT('Origin',(3.79999957308174,7.29999999999998,30.799999999963));
#145636=CARTESIAN_POINT('Origin',(3.89999957308174,10.6,14.1499999999815));
#145637=CARTESIAN_POINT('',(3.79999957308174,10.5,27.799999999963));
#145638=CARTESIAN_POINT('',(3.79999957308174,10.5,27.799999999963));
#145639=CARTESIAN_POINT('',(3.79999957308174,10.5,14.1499999999815));
#145640=CARTESIAN_POINT('Origin',(3.89999957308174,7.29999999999999,27.799999999963));
#145641=CARTESIAN_POINT('',(3.79999957308174,4.09999999999999,27.799999999963));
#145642=CARTESIAN_POINT('',(3.79999957308174,4.09999999999999,27.799999999963));
#145643=CARTESIAN_POINT('Origin',(3.79999957308174,7.29999999999999,27.799999999963));
#145644=CARTESIAN_POINT('Origin',(3.89999957308174,3.99999999999999,12.6499999999815));
#145645=CARTESIAN_POINT('',(3.79999957308174,4.09999999999999,12.6499999999815));
#145646=CARTESIAN_POINT('Origin',(3.99999957308175,10.5,30.799999999963));
#145647=CARTESIAN_POINT('',(1.99999957308175,10.5,30.799999999963));
#145648=CARTESIAN_POINT('',(3.99999957308175,10.5,30.799999999963));
#145649=CARTESIAN_POINT('',(1.99999957308175,10.5,27.799999999963));
#145650=CARTESIAN_POINT('',(1.99999957308175,10.5,27.799999999963));
#145651=CARTESIAN_POINT('',(3.99999957308175,10.5,27.799999999963));
#145652=CARTESIAN_POINT('Origin',(3.99999957308175,7.29999999999998,30.799999999963));
#145653=CARTESIAN_POINT('',(1.99999957308175,4.09999999999998,30.799999999963));
#145654=CARTESIAN_POINT('',(3.99999957308175,4.09999999999998,30.799999999963));
#145655=CARTESIAN_POINT('Origin',(1.99999957308175,7.29999999999998,30.799999999963));
#145656=CARTESIAN_POINT('Origin',(3.99999957308175,4.09999999999999,27.799999999963));
#145657=CARTESIAN_POINT('',(1.99999957308175,4.09999999999999,27.799999999963));
#145658=CARTESIAN_POINT('',(3.99999957308175,4.09999999999999,27.799999999963));
#145659=CARTESIAN_POINT('',(1.99999957308175,4.09999999999998,30.799999999963));
#145660=CARTESIAN_POINT('Origin',(3.99999957308175,7.29999999999999,27.799999999963));
#145661=CARTESIAN_POINT('Origin',(1.99999957308175,7.29999999999999,27.799999999963));
#145662=CARTESIAN_POINT('Origin',(1.99999957308175,7.29999999999999,29.299999999963));
#145663=CARTESIAN_POINT('',(1.99999957308175,8.99999999999999,27.799999999963));
#145664=CARTESIAN_POINT('',(1.99999957308174,8.99999999999999,30.049999999963));
#145665=CARTESIAN_POINT('',(1.99999957308175,5.59999999999999,27.799999999963));
#145666=CARTESIAN_POINT('Origin',(1.99999957308175,7.29999999999999,27.799999999963));
#145667=CARTESIAN_POINT('',(1.99999957308174,5.59999999999999,28.549999999963));
#145668=CARTESIAN_POINT('Origin',(3.99999957308175,8.99999999999998,30.799999999963));
#145669=CARTESIAN_POINT('',(3.99999957308175,8.99999999999999,27.799999999963));
#145670=CARTESIAN_POINT('Origin',(3.99999957308175,5.59999999999999,27.799999999963));
#145671=CARTESIAN_POINT('',(3.99999957308175,5.59999999999999,27.799999999963));
#145672=CARTESIAN_POINT('Origin',(3.99999957308175,7.29999999999999,27.799999999963));
#145673=CARTESIAN_POINT('Origin',(-5.84999999999999,14.85,12.049999999963));
#145674=CARTESIAN_POINT('',(-6.74999999999999,14.7121310205014,7.55127331643961));
#145675=CARTESIAN_POINT('Ctrl Pts',(-6.74999999999999,14.7121310205014,
7.5512733164396));
#145676=CARTESIAN_POINT('Ctrl Pts',(-6.59752601769717,14.6667024782955,
7.47444117971334));
#145677=CARTESIAN_POINT('Ctrl Pts',(-6.45066441870419,14.6042854333858,
7.39054870820519));
#145678=CARTESIAN_POINT('Ctrl Pts',(-6.23747959335272,14.4896253048058,
7.25461326047292));
#145679=CARTESIAN_POINT('Ctrl Pts',(-6.16538230807449,14.4461506137646,
7.20587149527676));
#145680=CARTESIAN_POINT('Ctrl Pts',(-6.0957241205081,14.4,7.15616513795545));
#145681=CARTESIAN_POINT('',(-7.94554708839804,15.3,8.64284834494288));
#145682=CARTESIAN_POINT('Ctrl Pts',(-6.74999999999999,14.7121310205014,
7.55127331643961));
#145683=CARTESIAN_POINT('Ctrl Pts',(-7.00710332219316,14.788733132856,7.68082851861365));
#145684=CARTESIAN_POINT('Ctrl Pts',(-7.24069578776386,14.8797238094481,
7.84718696018165));
#145685=CARTESIAN_POINT('Ctrl Pts',(-7.62292890725893,15.0675098561581,
8.1991278933308));
#145686=CARTESIAN_POINT('Ctrl Pts',(-7.80142030539744,15.1786537405669,
8.4117434285975));
#145687=CARTESIAN_POINT('Ctrl Pts',(-7.94554708839804,15.3,8.64284834494288));
#145688=CARTESIAN_POINT('',(-7.59791508502123,15.3,15.6478872766235));
#145689=CARTESIAN_POINT('Origin',(-5.84999999999999,15.3,12.049999999963));
#145690=CARTESIAN_POINT('Ctrl Pts',(-7.59791508502124,15.3,15.6478872766235));
#145691=CARTESIAN_POINT('Ctrl Pts',(-7.52392855362119,15.2606953607031,
15.7275286632141));
#145692=CARTESIAN_POINT('Ctrl Pts',(-7.4466010458344,15.2236063588331,15.8020015711092));
#145693=CARTESIAN_POINT('Ctrl Pts',(-7.17008331211839,15.1023689555337,
16.0423295793347));
#145694=CARTESIAN_POINT('Ctrl Pts',(-6.92898212028428,15.0179793780072,
16.2033520572508));
#145695=CARTESIAN_POINT('Ctrl Pts',(-6.56497369958393,14.9197507369652,
16.372867478824));
#145696=CARTESIAN_POINT('Ctrl Pts',(-6.4603790510634,14.8942778184954,16.4146017054756));
#145697=CARTESIAN_POINT('Ctrl Pts',(-6.35454545129335,14.8710452666677,
16.4501220343486));
#145698=CARTESIAN_POINT('Origin',(-5.84999999999999,-0.250000000000012,
12.049999999963));
#145699=CARTESIAN_POINT('',(-6.7499999280398,-0.112130999061391,7.55127328017863));
#145700=CARTESIAN_POINT('Ctrl Pts',(-6.0957241205081,0.199999999999987,
7.15616513795545));
#145701=CARTESIAN_POINT('Ctrl Pts',(-6.16538230807449,0.153849386235404,
7.20587149527676));
#145702=CARTESIAN_POINT('Ctrl Pts',(-6.23747959335272,0.110374695194135,
7.25461326047291));
#145703=CARTESIAN_POINT('Ctrl Pts',(-6.45066439686828,-0.00428542164149448,
7.39054869428171));
#145704=CARTESIAN_POINT('Ctrl Pts',(-6.59752597145899,-0.0667024587113867,
7.47444115333255));
#145705=CARTESIAN_POINT('Ctrl Pts',(-6.7499999280398,-0.112130999061384,
7.55127328017863));
#145706=CARTESIAN_POINT('',(-6.35454550078494,-0.271045277532096,16.450122017738));
#145707=CARTESIAN_POINT('Ctrl Pts',(-6.35454550078344,-0.271045277531764,
16.4501220177385));
#145708=CARTESIAN_POINT('Ctrl Pts',(-6.0567466526599,-0.205672592100444,
16.5500705489484));
#145709=CARTESIAN_POINT('Ctrl Pts',(-5.76835567822078,-0.0899428765078181,
16.6667013016116));
#145710=CARTESIAN_POINT('Ctrl Pts',(-5.41464812969736,0.102033642101067,
16.8329226337617));
#145711=CARTESIAN_POINT('Ctrl Pts',(-5.33338146986815,0.149875808238858,
16.8728497987674));
#145712=CARTESIAN_POINT('Ctrl Pts',(-5.25380888164336,0.199999999999991,
16.9135949821128));
#145713=CARTESIAN_POINT('',(-7.59791508502123,-0.700000000000012,15.6478872766235));
#145714=CARTESIAN_POINT('Ctrl Pts',(-6.35454550078494,-0.271045277532095,
16.450122017738));
#145715=CARTESIAN_POINT('Ctrl Pts',(-6.46037908367833,-0.294277826431993,
16.4146016924801));
#145716=CARTESIAN_POINT('Ctrl Pts',(-6.56497371540389,-0.319750741234298,
16.3728674714568));
#145717=CARTESIAN_POINT('Ctrl Pts',(-6.92898212028428,-0.417979378007196,
16.2033520572508));
#145718=CARTESIAN_POINT('Ctrl Pts',(-7.17008331211839,-0.502368955533736,
16.0423295793347));
#145719=CARTESIAN_POINT('Ctrl Pts',(-7.4466010458344,-0.623606358833087,
15.8020015711092));
#145720=CARTESIAN_POINT('Ctrl Pts',(-7.52392855362119,-0.660695360703133,
15.7275286632141));
#145721=CARTESIAN_POINT('Ctrl Pts',(-7.59791508502124,-0.700000000000011,
15.6478872766235));
#145722=CARTESIAN_POINT('',(-7.94554708839804,-0.700000000000012,8.64284834494287));
#145723=CARTESIAN_POINT('Origin',(-5.84999999999999,-0.700000000000012,
12.049999999963));
#145724=CARTESIAN_POINT('Ctrl Pts',(-7.94554708839804,-0.70000000000001,
8.64284834494287));
#145725=CARTESIAN_POINT('Ctrl Pts',(-7.80142030539744,-0.578653740566923,
8.4117434285975));
#145726=CARTESIAN_POINT('Ctrl Pts',(-7.62292890725893,-0.467509856158084,
8.1991278933308));
#145727=CARTESIAN_POINT('Ctrl Pts',(-7.24069576991161,-0.279723800677587,
7.8471869437442));
#145728=CARTESIAN_POINT('Ctrl Pts',(-7.00710327840368,-0.188733116017182,
7.68082848788949));
#145729=CARTESIAN_POINT('Ctrl Pts',(-6.7499999280464,-0.112130999063354,
7.55127328018196));
#145730=CARTESIAN_POINT('Origin',(-5.12499999999999,15.3,12.049999999963));
#145731=CARTESIAN_POINT('',(-8.39999999999999,15.3,10.2303589813634));
#145732=CARTESIAN_POINT('',(-8.39999999999999,15.3,13.6060329039916));
#145733=CARTESIAN_POINT('',(-8.39999999999999,15.3,11.1401794906632));
#145734=CARTESIAN_POINT('Origin',(-5.39999999999998,15.3,13.6060329039916));
#145735=CARTESIAN_POINT('Origin',(-5.4,15.3,10.2303589813634));
#145736=CARTESIAN_POINT('',(-4.34999999999999,15.3,12.049999999963));
#145737=CARTESIAN_POINT('Origin',(-5.84999999999999,15.3,12.049999999963));
#145738=CARTESIAN_POINT('Origin',(-5.12499999999999,-0.700000000000012,
12.049999999963));
#145739=CARTESIAN_POINT('',(-8.39999999999999,-0.700000000000012,13.6060329039916));
#145740=CARTESIAN_POINT('Origin',(-5.39999999999998,-0.700000000000012,
13.6060329039916));
#145741=CARTESIAN_POINT('',(-8.39999999999999,-0.700000000000012,10.2303589813634));
#145742=CARTESIAN_POINT('',(-8.39999999999999,-0.700000000000012,12.8280164519773));
#145743=CARTESIAN_POINT('Origin',(-5.4,-0.700000000000012,10.2303589813634));
#145744=CARTESIAN_POINT('',(-4.34999999999999,-0.700000000000012,12.049999999963));
#145745=CARTESIAN_POINT('Origin',(-5.84999999999999,-0.700000000000012,
12.049999999963));
#145746=CARTESIAN_POINT('Origin',(-5.84999999999999,2.19999999999999,12.049999999963));
#145747=CARTESIAN_POINT('',(-7.94554708839804,2.3,8.64284834494287));
#145748=CARTESIAN_POINT('Ctrl Pts',(-7.6638591912008,2.09999999999999,8.26187185607765));
#145749=CARTESIAN_POINT('Ctrl Pts',(-7.76664216185284,2.16222477820042,
8.38007744138255));
#145750=CARTESIAN_POINT('Ctrl Pts',(-7.86173330152362,2.22943372970385,
8.50845432184085));
#145751=CARTESIAN_POINT('Ctrl Pts',(-7.94554708839804,2.29999999999999,
8.64284834494287));
#145752=CARTESIAN_POINT('',(-7.59791508502123,2.29999999999999,15.6478872766235));
#145753=CARTESIAN_POINT('Origin',(-5.84999999999999,2.29999999999999,12.049999999963));
#145754=CARTESIAN_POINT('Ctrl Pts',(-7.59791508502124,2.29999999999999,
15.6478872766235));
#145755=CARTESIAN_POINT('Ctrl Pts',(-7.52392855362119,2.26069536070311,
15.7275286632141));
#145756=CARTESIAN_POINT('Ctrl Pts',(-7.4466010458344,2.22360635883307,15.8020015711092));
#145757=CARTESIAN_POINT('Ctrl Pts',(-7.29927642305898,2.15901283541843,
15.9300448350199));
#145758=CARTESIAN_POINT('Ctrl Pts',(-7.2255360033652,2.12910947683608,15.9886060423839));
#145759=CARTESIAN_POINT('Ctrl Pts',(-7.1474157554001,2.09999999999999,16.0445853799042));
#145760=CARTESIAN_POINT('Origin',(-5.84999999999999,11.8,12.049999999963));
#145761=CARTESIAN_POINT('',(-7.59791508502123,11.7,15.6478872766235));
#145762=CARTESIAN_POINT('Ctrl Pts',(-7.1474157554001,11.9,16.0445853799042));
#145763=CARTESIAN_POINT('Ctrl Pts',(-7.2255360033652,11.8708905231639,15.9886060423839));
#145764=CARTESIAN_POINT('Ctrl Pts',(-7.29927642305897,11.8409871645816,
15.9300448350199));
#145765=CARTESIAN_POINT('Ctrl Pts',(-7.4466010458344,11.7763936411669,15.8020015711092));
#145766=CARTESIAN_POINT('Ctrl Pts',(-7.52392855362119,11.7393046392969,
15.7275286632141));
#145767=CARTESIAN_POINT('Ctrl Pts',(-7.59791508502124,11.7,15.6478872766235));
#145768=CARTESIAN_POINT('',(-7.94554708839804,11.7,8.64284834494287));
#145769=CARTESIAN_POINT('Origin',(-5.84999999999999,11.7,12.049999999963));
#145770=CARTESIAN_POINT('Ctrl Pts',(-7.94554708839804,11.7,8.64284834494287));
#145771=CARTESIAN_POINT('Ctrl Pts',(-7.86174205772034,11.7705588980944,
8.50846836225769));
#145772=CARTESIAN_POINT('Ctrl Pts',(-7.76664825426621,11.8377715334544,
8.38008444796432));
#145773=CARTESIAN_POINT('Ctrl Pts',(-7.66385919120079,11.9,8.26187185607765));
#145774=CARTESIAN_POINT('Origin',(-5.12499999999999,11.7,12.049999999963));
#145775=CARTESIAN_POINT('',(-8.39999999999999,11.7,13.6060329039916));
#145776=CARTESIAN_POINT('',(-8.39999999999999,11.7,10.2303589813634));
#145777=CARTESIAN_POINT('',(-8.39999999999999,11.7,11.1401794906632));
#145778=CARTESIAN_POINT('Origin',(-5.4,11.7,10.2303589813634));
#145779=CARTESIAN_POINT('Origin',(-5.39999999999998,11.7,13.6060329039916));
#145780=CARTESIAN_POINT('',(-4.34999999999999,11.7,12.049999999963));
#145781=CARTESIAN_POINT('Origin',(-5.84999999999999,11.7,12.049999999963));
#145782=CARTESIAN_POINT('Origin',(-5.12499999999999,2.29999999999999,12.049999999963));
#145783=CARTESIAN_POINT('',(-8.39999999999999,2.29999999999999,13.6060329039916));
#145784=CARTESIAN_POINT('Origin',(-5.39999999999998,2.29999999999999,13.6060329039916));
#145785=CARTESIAN_POINT('',(-8.39999999999999,2.29999999999999,10.2303589813634));
#145786=CARTESIAN_POINT('Origin',(-5.4,2.29999999999999,10.2303589813634));
#145787=CARTESIAN_POINT('',(-8.39999999999999,2.29999999999999,13.6060329039916));
#145788=CARTESIAN_POINT('',(-4.34999999999999,2.29999999999999,12.049999999963));
#145789=CARTESIAN_POINT('Origin',(-5.84999999999999,2.29999999999999,12.049999999963));
#145790=CARTESIAN_POINT('Origin',(-8.89999999999999,14.4,24.0343597112987));
#145791=CARTESIAN_POINT('',(-6.35454545454544,14.4,16.4501220332571));
#145792=CARTESIAN_POINT('Origin',(-5.39999999999999,14.4,10.2303589813634));
#145793=CARTESIAN_POINT('',(-8.39999999999999,14.4,10.2303589813634));
#145794=CARTESIAN_POINT('',(-6.74999999999999,14.4,7.55127331643961));
#145795=CARTESIAN_POINT('Origin',(-8.39999999999999,14.4,16.049999999963));
#145796=CARTESIAN_POINT('',(-8.39999999999999,11.9,13.6060329039916));
#145797=CARTESIAN_POINT('Origin',(-5.39999999999999,14.4,13.6060329039916));
#145798=CARTESIAN_POINT('Origin',(1.33226762955019E-14,0.0999999999999934,
-4.44089209850063E-15));
#145799=CARTESIAN_POINT('',(4.00000000000001,0.0999999999999934,-4.44089209850063E-15));
#145800=CARTESIAN_POINT('Origin',(1.33226762955019E-14,0.0999999999999934,
-4.44089209850063E-15));
#145801=CARTESIAN_POINT('',(1.60000000000001,0.0999999999999934,-4.44089209850063E-15));
#145802=CARTESIAN_POINT('Origin',(1.33226762955019E-14,0.0999999999999934,
-4.44089209850063E-15));
#145803=CARTESIAN_POINT('Origin',(-2.20000021345912,0.199999999999987,17.0249999999815));
#145804=CARTESIAN_POINT('',(1.75280925781799,0.199999999999987,-3.59550548681377));
#145805=CARTESIAN_POINT('Origin',(1.33226762955019E-14,0.199999999999991,
-4.44089209850063E-15));
#145806=CARTESIAN_POINT('',(4.21701869329868,0.199999999999991,-2.3942031587951));
#145807=CARTESIAN_POINT('Origin',(1.33226762955019E-14,14.5,-4.44089209850063E-15));
#145808=CARTESIAN_POINT('',(4.00000000000001,14.5,-4.44089209850063E-15));
#145809=CARTESIAN_POINT('Origin',(1.33226762955019E-14,14.5,-4.44089209850063E-15));
#145810=CARTESIAN_POINT('',(1.60000000000001,14.5,-4.44089209850063E-15));
#145811=CARTESIAN_POINT('Origin',(1.33226762955019E-14,14.5,-4.44089209850063E-15));
#145812=CARTESIAN_POINT('Origin',(-2.20000021345912,14.4,17.0249999999815));
#145813=CARTESIAN_POINT('',(1.75280925781799,14.4,-3.59550548681377));
#145814=CARTESIAN_POINT('Origin',(1.33226762955019E-14,14.4,-4.44089209850063E-15));
#145815=CARTESIAN_POINT('',(3.99999957308175,14.4,-2.5));
#145816=CARTESIAN_POINT('Origin',(-3.99999999999999,14.4,8.04999999996301));
#145817=CARTESIAN_POINT('',(-3.99999999999999,14.4,-4.44089209850063E-15));
#145818=CARTESIAN_POINT('',(-3.99999999999999,14.4,3.08613054156667));
#145819=CARTESIAN_POINT('Origin',(-8.39999999999999,14.4,16.049999999963));
#145820=CARTESIAN_POINT('',(-8.39999999999999,14.4,10.2303589813634));
#145821=CARTESIAN_POINT('',(-8.39999999999999,14.4,13.6060329039916));
#145822=CARTESIAN_POINT('Origin',(-8.99999999999999,14.4,3.08613054156667));
#145823=CARTESIAN_POINT('Origin',(-8.99999999999999,14.4,3.08613054156667));
#145824=CARTESIAN_POINT('',(-6.74999999999999,14.4,7.55127331643961));
#145825=CARTESIAN_POINT('Origin',(-5.39999999999999,14.4,10.2303589813634));
#145826=CARTESIAN_POINT('Origin',(-5.84999999999999,14.4,12.049999999963));
#145827=CARTESIAN_POINT('',(-4.34999999999999,14.4,12.049999999963));
#145828=CARTESIAN_POINT('Origin',(-5.39999999999999,14.4,13.6060329039916));
#145829=CARTESIAN_POINT('Origin',(3.99999957308175,14.4,38.299999999963));
#145830=CARTESIAN_POINT('Origin',(1.75280925781799,14.4,-3.59550548681377));
#145831=CARTESIAN_POINT('',(1.75280925781799,14.4,-3.59550548681377));
#145832=CARTESIAN_POINT('Origin',(1.33226762955019E-14,14.4,-4.44089209850063E-15));
#145833=CARTESIAN_POINT('',(1.60000000000001,14.4,-4.24494861063705E-15));
#145834=CARTESIAN_POINT('Origin',(-5.84999999999999,14.4,12.049999999963));
#145835=CARTESIAN_POINT('',(-4.34999999999999,14.4,12.049999999963));
#145836=CARTESIAN_POINT('Origin',(1.33226762955019E-14,14.4,-4.44089209850063E-15));
#145837=CARTESIAN_POINT('',(4.00000000000001,14.4,-3.95103337884168E-15));
#145838=CARTESIAN_POINT('',(4.00000000000001,14.4,-3.95103337884168E-15));
#459196=UNCERTAINTY_MEASURE_WITH_UNIT(LENGTH_MEASURE(0.01),#459243,
'DISTANCE_ACCURACY_VALUE',
'Maximum model space distance between geometric entities at asserted c
onnectivities');
#459216=UNCERTAINTY_MEASURE_WITH_UNIT(LENGTH_MEASURE(0.01),#459243,
'DISTANCE_ACCURACY_VALUE',
'Maximum model space distance between geometric entities at asserted c
onnectivities');
#459222=(
GEOMETRIC_REPRESENTATION_CONTEXT(3)
GLOBAL_UNCERTAINTY_ASSIGNED_CONTEXT((#459196))
GLOBAL_UNIT_ASSIGNED_CONTEXT((#459243,#459245,#459246))
REPRESENTATION_CONTEXT('','3D')
);
#459242=(
GEOMETRIC_REPRESENTATION_CONTEXT(3)
GLOBAL_UNCERTAINTY_ASSIGNED_CONTEXT((#459216))
GLOBAL_UNIT_ASSIGNED_CONTEXT((#459243,#459245,#459246))
REPRESENTATION_CONTEXT('','3D')
);
#459243=(
LENGTH_UNIT()
NAMED_UNIT(*)
SI_UNIT(.MILLI.,.METRE.)
);
#459245=(
NAMED_UNIT(*)
PLANE_ANGLE_UNIT()
SI_UNIT($,.RADIAN.)
);
#459246=(
NAMED_UNIT(*)
SI_UNIT($,.STERADIAN.)
SOLID_ANGLE_UNIT()
);
#459252=SHAPE_DEFINITION_REPRESENTATION(#459277,#459333);
#459277=PRODUCT_DEFINITION_SHAPE('',$,#459359);
#459333=SHAPE_REPRESENTATION('',(#97093),#459222);
#459353=PRODUCT_DEFINITION_CONTEXT('part definition',#459430,'design');
#459359=PRODUCT_DEFINITION('Tension Rocker Arm','Tension Rocker Arm',#459384,
#459353);
#459384=PRODUCT_DEFINITION_FORMATION('',$,#459437);
#459430=APPLICATION_CONTEXT(
'Core Data for Automotive Mechanical Design Process');
#459431=PRODUCT_CONTEXT('part definition',#459430,'mechanical');
#459437=PRODUCT('Tension Rocker Arm','Tension Rocker Arm',$,(#459431));
#459513=COLOUR_RGB('Sky Blue',0.24,0.69,0.87);
#459514=FILL_AREA_STYLE_COLOUR('',#459513);
#459515=FILL_AREA_STYLE('',(#459514));
#459516=SURFACE_STYLE_FILL_AREA(#459515);
#459517=SURFACE_SIDE_STYLE('',(#459516));
#459518=SURFACE_STYLE_USAGE(.BOTH.,#459517);
#459519=PRESENTATION_STYLE_ASSIGNMENT((#459518));
ENDSEC;
END-ISO-10303-21;
